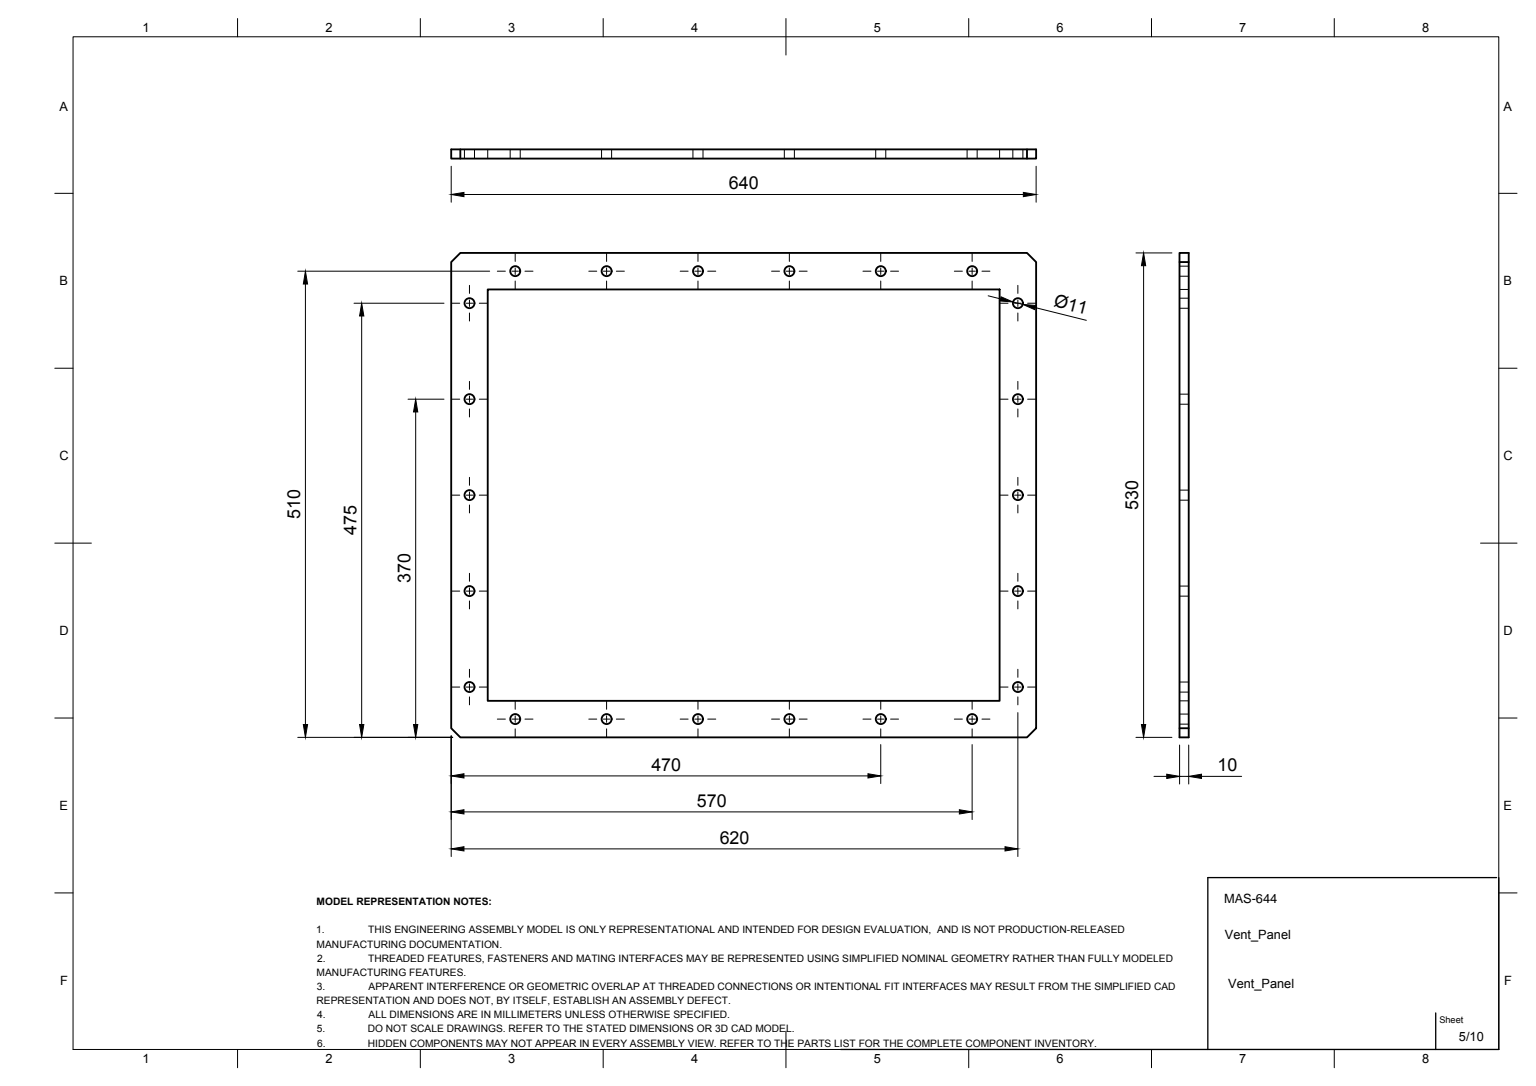
ISO-10303-21;
HEADER;
FILE_DESCRIPTION((''),'2;1');
FILE_NAME('Vent_Panel.step','2026-10-09T11:38:21-07:00',(''),(''),'','','');
FILE_SCHEMA (('AUTOMOTIVE_DESIGN { 1 0 10303 214 3 1 1 }'));
ENDSEC;
DATA;
#10=MECHANICAL_DESIGN_GEOMETRIC_PRESENTATION_REPRESENTATION('',(#61),#3619);
#45=SHAPE_REPRESENTATION_RELATIONSHIP('SRR','None',#3653,#53) ;
#53=ADVANCED_BREP_SHAPE_REPRESENTATION('',(#69),#3613) ;
#61=STYLED_ITEM('',(#3700),#69) ;
#69=MANIFOLD_SOLID_BREP('Body1',#2085) ;
#111=FACE_BOUND('',#414,.T.) ;
#112=FACE_BOUND('',#415,.T.) ;
#113=FACE_BOUND('',#416,.T.) ;
#114=FACE_BOUND('',#417,.T.) ;
#115=FACE_BOUND('',#418,.T.) ;
#116=FACE_BOUND('',#419,.T.) ;
#117=FACE_BOUND('',#420,.T.) ;
#118=FACE_BOUND('',#421,.T.) ;
#119=FACE_BOUND('',#422,.T.) ;
#120=FACE_BOUND('',#423,.T.) ;
#121=FACE_BOUND('',#424,.T.) ;
#122=FACE_BOUND('',#425,.T.) ;
#123=FACE_BOUND('',#426,.T.) ;
#124=FACE_BOUND('',#427,.T.) ;
#125=FACE_BOUND('',#428,.T.) ;
#126=FACE_BOUND('',#429,.T.) ;
#127=FACE_BOUND('',#430,.T.) ;
#128=FACE_BOUND('',#431,.T.) ;
#129=FACE_BOUND('',#432,.T.) ;
#130=FACE_BOUND('',#433,.T.) ;
#131=FACE_BOUND('',#434,.T.) ;
#132=FACE_BOUND('',#435,.T.) ;
#133=FACE_BOUND('',#436,.T.) ;
#134=FACE_BOUND('',#438,.T.) ;
#135=FACE_BOUND('',#439,.T.) ;
#136=FACE_BOUND('',#440,.T.) ;
#137=FACE_BOUND('',#441,.T.) ;
#138=FACE_BOUND('',#442,.T.) ;
#139=FACE_BOUND('',#443,.T.) ;
#140=FACE_BOUND('',#444,.T.) ;
#141=FACE_BOUND('',#445,.T.) ;
#142=FACE_BOUND('',#446,.T.) ;
#143=FACE_BOUND('',#447,.T.) ;
#144=FACE_BOUND('',#448,.T.) ;
#145=FACE_BOUND('',#449,.T.) ;
#146=FACE_BOUND('',#450,.T.) ;
#147=FACE_BOUND('',#451,.T.) ;
#148=FACE_BOUND('',#452,.T.) ;
#149=FACE_BOUND('',#453,.T.) ;
#150=FACE_BOUND('',#454,.T.) ;
#151=FACE_BOUND('',#455,.T.) ;
#152=FACE_BOUND('',#456,.T.) ;
#153=FACE_BOUND('',#457,.T.) ;
#154=FACE_BOUND('',#458,.T.) ;
#155=FACE_BOUND('',#459,.T.) ;
#156=FACE_BOUND('',#460,.T.) ;
#169=PLANE('',#2328) ;
#170=PLANE('',#2329) ;
#171=PLANE('',#2330) ;
#172=PLANE('',#2331) ;
#173=PLANE('',#2332) ;
#174=PLANE('',#2333) ;
#175=PLANE('',#2334) ;
#176=PLANE('',#2335) ;
#177=PLANE('',#2336) ;
#178=PLANE('',#2337) ;
#179=PLANE('',#2338) ;
#180=PLANE('',#2339) ;
#181=PLANE('',#2340) ;
#182=PLANE('',#2341) ;
#247=FACE_OUTER_BOUND('',#391,.T.) ;
#248=FACE_OUTER_BOUND('',#392,.T.) ;
#249=FACE_OUTER_BOUND('',#393,.T.) ;
#250=FACE_OUTER_BOUND('',#394,.T.) ;
#251=FACE_OUTER_BOUND('',#395,.T.) ;
#252=FACE_OUTER_BOUND('',#396,.T.) ;
#253=FACE_OUTER_BOUND('',#397,.T.) ;
#254=FACE_OUTER_BOUND('',#398,.T.) ;
#255=FACE_OUTER_BOUND('',#399,.T.) ;
#256=FACE_OUTER_BOUND('',#400,.T.) ;
#257=FACE_OUTER_BOUND('',#401,.T.) ;
#258=FACE_OUTER_BOUND('',#402,.T.) ;
#259=FACE_OUTER_BOUND('',#403,.T.) ;
#260=FACE_OUTER_BOUND('',#404,.T.) ;
#261=FACE_OUTER_BOUND('',#405,.T.) ;
#262=FACE_OUTER_BOUND('',#406,.T.) ;
#263=FACE_OUTER_BOUND('',#407,.T.) ;
#264=FACE_OUTER_BOUND('',#408,.T.) ;
#265=FACE_OUTER_BOUND('',#409,.T.) ;
#266=FACE_OUTER_BOUND('',#410,.T.) ;
#267=FACE_OUTER_BOUND('',#411,.T.) ;
#268=FACE_OUTER_BOUND('',#412,.T.) ;
#269=FACE_OUTER_BOUND('',#413,.T.) ;
#270=FACE_OUTER_BOUND('',#437,.T.) ;
#271=FACE_OUTER_BOUND('',#461,.T.) ;
#272=FACE_OUTER_BOUND('',#462,.T.) ;
#273=FACE_OUTER_BOUND('',#463,.T.) ;
#274=FACE_OUTER_BOUND('',#464,.T.) ;
#275=FACE_OUTER_BOUND('',#465,.T.) ;
#276=FACE_OUTER_BOUND('',#466,.T.) ;
#277=FACE_OUTER_BOUND('',#467,.T.) ;
#278=FACE_OUTER_BOUND('',#468,.T.) ;
#279=FACE_OUTER_BOUND('',#469,.T.) ;
#280=FACE_OUTER_BOUND('',#470,.T.) ;
#281=FACE_OUTER_BOUND('',#471,.T.) ;
#282=FACE_OUTER_BOUND('',#472,.T.) ;
#391=EDGE_LOOP('',(#1567,#1568,#1569,#1570)) ;
#392=EDGE_LOOP('',(#1571,#1572,#1573,#1574)) ;
#393=EDGE_LOOP('',(#1575,#1576,#1577,#1578)) ;
#394=EDGE_LOOP('',(#1579,#1580,#1581,#1582)) ;
#395=EDGE_LOOP('',(#1583,#1584,#1585,#1586)) ;
#396=EDGE_LOOP('',(#1587,#1588,#1589,#1590)) ;
#397=EDGE_LOOP('',(#1591,#1592,#1593,#1594)) ;
#398=EDGE_LOOP('',(#1595,#1596,#1597,#1598)) ;
#399=EDGE_LOOP('',(#1599,#1600,#1601,#1602)) ;
#400=EDGE_LOOP('',(#1603,#1604,#1605,#1606)) ;
#401=EDGE_LOOP('',(#1607,#1608,#1609,#1610)) ;
#402=EDGE_LOOP('',(#1611,#1612,#1613,#1614)) ;
#403=EDGE_LOOP('',(#1615,#1616,#1617,#1618)) ;
#404=EDGE_LOOP('',(#1619,#1620,#1621,#1622)) ;
#405=EDGE_LOOP('',(#1623,#1624,#1625,#1626)) ;
#406=EDGE_LOOP('',(#1627,#1628,#1629,#1630)) ;
#407=EDGE_LOOP('',(#1631,#1632,#1633,#1634)) ;
#408=EDGE_LOOP('',(#1635,#1636,#1637,#1638)) ;
#409=EDGE_LOOP('',(#1639,#1640,#1641,#1642)) ;
#410=EDGE_LOOP('',(#1643,#1644,#1645,#1646)) ;
#411=EDGE_LOOP('',(#1647,#1648,#1649,#1650)) ;
#412=EDGE_LOOP('',(#1651,#1652,#1653,#1654)) ;
#413=EDGE_LOOP('',(#1655,#1656,#1657,#1658,#1659,#1660,#1661,#1662)) ;
#414=EDGE_LOOP('',(#1663,#1664,#1665,#1666)) ;
#415=EDGE_LOOP('',(#1667)) ;
#416=EDGE_LOOP('',(#1668)) ;
#417=EDGE_LOOP('',(#1669)) ;
#418=EDGE_LOOP('',(#1670)) ;
#419=EDGE_LOOP('',(#1671)) ;
#420=EDGE_LOOP('',(#1672)) ;
#421=EDGE_LOOP('',(#1673)) ;
#422=EDGE_LOOP('',(#1674)) ;
#423=EDGE_LOOP('',(#1675)) ;
#424=EDGE_LOOP('',(#1676)) ;
#425=EDGE_LOOP('',(#1677)) ;
#426=EDGE_LOOP('',(#1678)) ;
#427=EDGE_LOOP('',(#1679)) ;
#428=EDGE_LOOP('',(#1680)) ;
#429=EDGE_LOOP('',(#1681)) ;
#430=EDGE_LOOP('',(#1682)) ;
#431=EDGE_LOOP('',(#1683)) ;
#432=EDGE_LOOP('',(#1684)) ;
#433=EDGE_LOOP('',(#1685)) ;
#434=EDGE_LOOP('',(#1686)) ;
#435=EDGE_LOOP('',(#1687)) ;
#436=EDGE_LOOP('',(#1688)) ;
#437=EDGE_LOOP('',(#1689,#1690,#1691,#1692,#1693,#1694,#1695,#1696)) ;
#438=EDGE_LOOP('',(#1697,#1698,#1699,#1700)) ;
#439=EDGE_LOOP('',(#1701)) ;
#440=EDGE_LOOP('',(#1702)) ;
#441=EDGE_LOOP('',(#1703)) ;
#442=EDGE_LOOP('',(#1704)) ;
#443=EDGE_LOOP('',(#1705)) ;
#444=EDGE_LOOP('',(#1706)) ;
#445=EDGE_LOOP('',(#1707)) ;
#446=EDGE_LOOP('',(#1708)) ;
#447=EDGE_LOOP('',(#1709)) ;
#448=EDGE_LOOP('',(#1710)) ;
#449=EDGE_LOOP('',(#1711)) ;
#450=EDGE_LOOP('',(#1712)) ;
#451=EDGE_LOOP('',(#1713)) ;
#452=EDGE_LOOP('',(#1714)) ;
#453=EDGE_LOOP('',(#1715)) ;
#454=EDGE_LOOP('',(#1716)) ;
#455=EDGE_LOOP('',(#1717)) ;
#456=EDGE_LOOP('',(#1718)) ;
#457=EDGE_LOOP('',(#1719)) ;
#458=EDGE_LOOP('',(#1720)) ;
#459=EDGE_LOOP('',(#1721)) ;
#460=EDGE_LOOP('',(#1722)) ;
#461=EDGE_LOOP('',(#1723,#1724,#1725,#1726)) ;
#462=EDGE_LOOP('',(#1727,#1728,#1729,#1730)) ;
#463=EDGE_LOOP('',(#1731,#1732,#1733,#1734)) ;
#464=EDGE_LOOP('',(#1735,#1736,#1737,#1738)) ;
#465=EDGE_LOOP('',(#1739,#1740,#1741,#1742)) ;
#466=EDGE_LOOP('',(#1743,#1744,#1745,#1746)) ;
#467=EDGE_LOOP('',(#1747,#1748,#1749,#1750)) ;
#468=EDGE_LOOP('',(#1751,#1752,#1753,#1754)) ;
#469=EDGE_LOOP('',(#1755,#1756,#1757,#1758)) ;
#470=EDGE_LOOP('',(#1759,#1760,#1761,#1762)) ;
#471=EDGE_LOOP('',(#1763,#1764,#1765,#1766)) ;
#472=EDGE_LOOP('',(#1767,#1768,#1769,#1770)) ;
#557=LINE('',#3223,#721) ;
#558=LINE('',#3229,#722) ;
#559=LINE('',#3235,#723) ;
#560=LINE('',#3241,#724) ;
#561=LINE('',#3247,#725) ;
#562=LINE('',#3253,#726) ;
#563=LINE('',#3259,#727) ;
#564=LINE('',#3265,#728) ;
#565=LINE('',#3271,#729) ;
#566=LINE('',#3277,#730) ;
#567=LINE('',#3283,#731) ;
#568=LINE('',#3289,#732) ;
#569=LINE('',#3295,#733) ;
#570=LINE('',#3301,#734) ;
#571=LINE('',#3307,#735) ;
#572=LINE('',#3313,#736) ;
#573=LINE('',#3319,#737) ;
#574=LINE('',#3325,#738) ;
#575=LINE('',#3331,#739) ;
#576=LINE('',#3337,#740) ;
#577=LINE('',#3343,#741) ;
#578=LINE('',#3349,#742) ;
#579=LINE('',#3354,#743) ;
#580=LINE('',#3356,#744) ;
#581=LINE('',#3358,#745) ;
#582=LINE('',#3360,#746) ;
#583=LINE('',#3362,#747) ;
#584=LINE('',#3364,#748) ;
#585=LINE('',#3366,#749) ;
#586=LINE('',#3367,#750) ;
#587=LINE('',#3370,#751) ;
#588=LINE('',#3372,#752) ;
#589=LINE('',#3374,#753) ;
#590=LINE('',#3375,#754) ;
#591=LINE('',#3379,#755) ;
#592=LINE('',#3381,#756) ;
#593=LINE('',#3383,#757) ;
#594=LINE('',#3385,#758) ;
#595=LINE('',#3387,#759) ;
#596=LINE('',#3389,#760) ;
#597=LINE('',#3391,#761) ;
#598=LINE('',#3392,#762) ;
#599=LINE('',#3395,#763) ;
#600=LINE('',#3397,#764) ;
#601=LINE('',#3399,#765) ;
#602=LINE('',#3400,#766) ;
#603=LINE('',#3402,#767) ;
#604=LINE('',#3403,#768) ;
#605=LINE('',#3405,#769) ;
#606=LINE('',#3407,#770) ;
#607=LINE('',#3409,#771) ;
#608=LINE('',#3411,#772) ;
#609=LINE('',#3413,#773) ;
#610=LINE('',#3415,#774) ;
#611=LINE('',#3418,#775) ;
#612=LINE('',#3419,#776) ;
#613=LINE('',#3421,#777) ;
#614=LINE('',#3423,#778) ;
#721=VECTOR('',#2623,5.50000000000002) ;
#722=VECTOR('',#2630,5.50000000000002) ;
#723=VECTOR('',#2637,5.50000000000001) ;
#724=VECTOR('',#2644,5.50000000000001) ;
#725=VECTOR('',#2651,5.50000000000001) ;
#726=VECTOR('',#2658,5.50000000000001) ;
#727=VECTOR('',#2665,5.50000000000001) ;
#728=VECTOR('',#2672,5.50000000000001) ;
#729=VECTOR('',#2679,5.50000000000002) ;
#730=VECTOR('',#2686,5.50000000000002) ;
#731=VECTOR('',#2693,5.49999999999999) ;
#732=VECTOR('',#2700,5.49999999999999) ;
#733=VECTOR('',#2707,5.49999999999999) ;
#734=VECTOR('',#2714,5.49999999999999) ;
#735=VECTOR('',#2721,5.49999999999999) ;
#736=VECTOR('',#2728,5.50000000000002) ;
#737=VECTOR('',#2735,5.50000000000001) ;
#738=VECTOR('',#2742,5.50000000000001) ;
#739=VECTOR('',#2749,5.50000000000001) ;
#740=VECTOR('',#2756,5.50000000000001) ;
#741=VECTOR('',#2763,5.50000000000001) ;
#742=VECTOR('',#2770,5.50000000000001) ;
#743=VECTOR('',#2775,1000.) ;
#744=VECTOR('',#2776,1000.) ;
#745=VECTOR('',#2777,1000.) ;
#746=VECTOR('',#2778,1000.) ;
#747=VECTOR('',#2779,1000.) ;
#748=VECTOR('',#2780,1000.) ;
#749=VECTOR('',#2781,1000.) ;
#750=VECTOR('',#2782,1000.) ;
#751=VECTOR('',#2783,1000.) ;
#752=VECTOR('',#2784,1000.) ;
#753=VECTOR('',#2785,1000.) ;
#754=VECTOR('',#2786,1000.) ;
#755=VECTOR('',#2789,1000.) ;
#756=VECTOR('',#2790,1000.) ;
#757=VECTOR('',#2791,1000.) ;
#758=VECTOR('',#2792,1000.) ;
#759=VECTOR('',#2793,1000.) ;
#760=VECTOR('',#2794,1000.) ;
#761=VECTOR('',#2795,1000.) ;
#762=VECTOR('',#2796,1000.) ;
#763=VECTOR('',#2797,1000.) ;
#764=VECTOR('',#2798,1000.) ;
#765=VECTOR('',#2799,1000.) ;
#766=VECTOR('',#2800,1000.) ;
#767=VECTOR('',#2803,1000.) ;
#768=VECTOR('',#2804,1000.) ;
#769=VECTOR('',#2807,1000.) ;
#770=VECTOR('',#2810,1000.) ;
#771=VECTOR('',#2813,1000.) ;
#772=VECTOR('',#2816,1000.) ;
#773=VECTOR('',#2819,1000.) ;
#774=VECTOR('',#2822,1000.) ;
#775=VECTOR('',#2827,1000.) ;
#776=VECTOR('',#2828,1000.) ;
#777=VECTOR('',#2831,1000.) ;
#778=VECTOR('',#2834,1000.) ;
#883=CIRCLE('',#2263,5.50000000000002) ;
#884=CIRCLE('',#2264,5.50000000000002) ;
#885=CIRCLE('',#2266,5.50000000000002) ;
#886=CIRCLE('',#2267,5.50000000000002) ;
#887=CIRCLE('',#2269,5.50000000000001) ;
#888=CIRCLE('',#2270,5.50000000000001) ;
#889=CIRCLE('',#2272,5.50000000000001) ;
#890=CIRCLE('',#2273,5.50000000000001) ;
#891=CIRCLE('',#2275,5.50000000000001) ;
#892=CIRCLE('',#2276,5.50000000000001) ;
#893=CIRCLE('',#2278,5.50000000000001) ;
#894=CIRCLE('',#2279,5.50000000000001) ;
#895=CIRCLE('',#2281,5.50000000000001) ;
#896=CIRCLE('',#2282,5.50000000000001) ;
#897=CIRCLE('',#2284,5.50000000000001) ;
#898=CIRCLE('',#2285,5.50000000000001) ;
#899=CIRCLE('',#2287,5.50000000000002) ;
#900=CIRCLE('',#2288,5.50000000000002) ;
#901=CIRCLE('',#2290,5.50000000000002) ;
#902=CIRCLE('',#2291,5.50000000000002) ;
#903=CIRCLE('',#2293,5.49999999999999) ;
#904=CIRCLE('',#2294,5.49999999999999) ;
#905=CIRCLE('',#2296,5.49999999999999) ;
#906=CIRCLE('',#2297,5.49999999999999) ;
#907=CIRCLE('',#2299,5.49999999999999) ;
#908=CIRCLE('',#2300,5.49999999999999) ;
#909=CIRCLE('',#2302,5.49999999999999) ;
#910=CIRCLE('',#2303,5.49999999999999) ;
#911=CIRCLE('',#2305,5.49999999999999) ;
#912=CIRCLE('',#2306,5.49999999999999) ;
#913=CIRCLE('',#2308,5.50000000000002) ;
#914=CIRCLE('',#2309,5.50000000000002) ;
#915=CIRCLE('',#2311,5.50000000000001) ;
#916=CIRCLE('',#2312,5.50000000000001) ;
#917=CIRCLE('',#2314,5.50000000000001) ;
#918=CIRCLE('',#2315,5.50000000000001) ;
#919=CIRCLE('',#2317,5.50000000000001) ;
#920=CIRCLE('',#2318,5.50000000000001) ;
#921=CIRCLE('',#2320,5.50000000000001) ;
#922=CIRCLE('',#2321,5.50000000000001) ;
#923=CIRCLE('',#2323,5.50000000000001) ;
#924=CIRCLE('',#2324,5.50000000000001) ;
#925=CIRCLE('',#2326,5.50000000000001) ;
#926=CIRCLE('',#2327,5.50000000000001) ;
#1003=VERTEX_POINT('',#3220) ;
#1004=VERTEX_POINT('',#3222) ;
#1005=VERTEX_POINT('',#3226) ;
#1006=VERTEX_POINT('',#3228) ;
#1007=VERTEX_POINT('',#3232) ;
#1008=VERTEX_POINT('',#3234) ;
#1009=VERTEX_POINT('',#3238) ;
#1010=VERTEX_POINT('',#3240) ;
#1011=VERTEX_POINT('',#3244) ;
#1012=VERTEX_POINT('',#3246) ;
#1013=VERTEX_POINT('',#3250) ;
#1014=VERTEX_POINT('',#3252) ;
#1015=VERTEX_POINT('',#3256) ;
#1016=VERTEX_POINT('',#3258) ;
#1017=VERTEX_POINT('',#3262) ;
#1018=VERTEX_POINT('',#3264) ;
#1019=VERTEX_POINT('',#3268) ;
#1020=VERTEX_POINT('',#3270) ;
#1021=VERTEX_POINT('',#3274) ;
#1022=VERTEX_POINT('',#3276) ;
#1023=VERTEX_POINT('',#3280) ;
#1024=VERTEX_POINT('',#3282) ;
#1025=VERTEX_POINT('',#3286) ;
#1026=VERTEX_POINT('',#3288) ;
#1027=VERTEX_POINT('',#3292) ;
#1028=VERTEX_POINT('',#3294) ;
#1029=VERTEX_POINT('',#3298) ;
#1030=VERTEX_POINT('',#3300) ;
#1031=VERTEX_POINT('',#3304) ;
#1032=VERTEX_POINT('',#3306) ;
#1033=VERTEX_POINT('',#3310) ;
#1034=VERTEX_POINT('',#3312) ;
#1035=VERTEX_POINT('',#3316) ;
#1036=VERTEX_POINT('',#3318) ;
#1037=VERTEX_POINT('',#3322) ;
#1038=VERTEX_POINT('',#3324) ;
#1039=VERTEX_POINT('',#3328) ;
#1040=VERTEX_POINT('',#3330) ;
#1041=VERTEX_POINT('',#3334) ;
#1042=VERTEX_POINT('',#3336) ;
#1043=VERTEX_POINT('',#3340) ;
#1044=VERTEX_POINT('',#3342) ;
#1045=VERTEX_POINT('',#3346) ;
#1046=VERTEX_POINT('',#3348) ;
#1047=VERTEX_POINT('',#3352) ;
#1048=VERTEX_POINT('',#3353) ;
#1049=VERTEX_POINT('',#3355) ;
#1050=VERTEX_POINT('',#3357) ;
#1051=VERTEX_POINT('',#3359) ;
#1052=VERTEX_POINT('',#3361) ;
#1053=VERTEX_POINT('',#3363) ;
#1054=VERTEX_POINT('',#3365) ;
#1055=VERTEX_POINT('',#3368) ;
#1056=VERTEX_POINT('',#3369) ;
#1057=VERTEX_POINT('',#3371) ;
#1058=VERTEX_POINT('',#3373) ;
#1059=VERTEX_POINT('',#3377) ;
#1060=VERTEX_POINT('',#3378) ;
#1061=VERTEX_POINT('',#3380) ;
#1062=VERTEX_POINT('',#3382) ;
#1063=VERTEX_POINT('',#3384) ;
#1064=VERTEX_POINT('',#3386) ;
#1065=VERTEX_POINT('',#3388) ;
#1066=VERTEX_POINT('',#3390) ;
#1067=VERTEX_POINT('',#3393) ;
#1068=VERTEX_POINT('',#3394) ;
#1069=VERTEX_POINT('',#3396) ;
#1070=VERTEX_POINT('',#3398) ;
#1209=EDGE_CURVE('',#1003,#1003,#883,.T.) ;
#1210=EDGE_CURVE('',#1003,#1004,#557,.T.) ;
#1211=EDGE_CURVE('',#1004,#1004,#884,.T.) ;
#1212=EDGE_CURVE('',#1005,#1005,#885,.T.) ;
#1213=EDGE_CURVE('',#1005,#1006,#558,.T.) ;
#1214=EDGE_CURVE('',#1006,#1006,#886,.T.) ;
#1215=EDGE_CURVE('',#1007,#1007,#887,.T.) ;
#1216=EDGE_CURVE('',#1007,#1008,#559,.T.) ;
#1217=EDGE_CURVE('',#1008,#1008,#888,.T.) ;
#1218=EDGE_CURVE('',#1009,#1009,#889,.T.) ;
#1219=EDGE_CURVE('',#1009,#1010,#560,.T.) ;
#1220=EDGE_CURVE('',#1010,#1010,#890,.T.) ;
#1221=EDGE_CURVE('',#1011,#1011,#891,.T.) ;
#1222=EDGE_CURVE('',#1011,#1012,#561,.T.) ;
#1223=EDGE_CURVE('',#1012,#1012,#892,.T.) ;
#1224=EDGE_CURVE('',#1013,#1013,#893,.T.) ;
#1225=EDGE_CURVE('',#1013,#1014,#562,.T.) ;
#1226=EDGE_CURVE('',#1014,#1014,#894,.T.) ;
#1227=EDGE_CURVE('',#1015,#1015,#895,.T.) ;
#1228=EDGE_CURVE('',#1015,#1016,#563,.T.) ;
#1229=EDGE_CURVE('',#1016,#1016,#896,.T.) ;
#1230=EDGE_CURVE('',#1017,#1017,#897,.T.) ;
#1231=EDGE_CURVE('',#1017,#1018,#564,.T.) ;
#1232=EDGE_CURVE('',#1018,#1018,#898,.T.) ;
#1233=EDGE_CURVE('',#1019,#1019,#899,.T.) ;
#1234=EDGE_CURVE('',#1019,#1020,#565,.T.) ;
#1235=EDGE_CURVE('',#1020,#1020,#900,.T.) ;
#1236=EDGE_CURVE('',#1021,#1021,#901,.T.) ;
#1237=EDGE_CURVE('',#1021,#1022,#566,.T.) ;
#1238=EDGE_CURVE('',#1022,#1022,#902,.T.) ;
#1239=EDGE_CURVE('',#1023,#1023,#903,.T.) ;
#1240=EDGE_CURVE('',#1023,#1024,#567,.T.) ;
#1241=EDGE_CURVE('',#1024,#1024,#904,.T.) ;
#1242=EDGE_CURVE('',#1025,#1025,#905,.T.) ;
#1243=EDGE_CURVE('',#1025,#1026,#568,.T.) ;
#1244=EDGE_CURVE('',#1026,#1026,#906,.T.) ;
#1245=EDGE_CURVE('',#1027,#1027,#907,.T.) ;
#1246=EDGE_CURVE('',#1027,#1028,#569,.T.) ;
#1247=EDGE_CURVE('',#1028,#1028,#908,.T.) ;
#1248=EDGE_CURVE('',#1029,#1029,#909,.T.) ;
#1249=EDGE_CURVE('',#1029,#1030,#570,.T.) ;
#1250=EDGE_CURVE('',#1030,#1030,#910,.T.) ;
#1251=EDGE_CURVE('',#1031,#1031,#911,.T.) ;
#1252=EDGE_CURVE('',#1031,#1032,#571,.T.) ;
#1253=EDGE_CURVE('',#1032,#1032,#912,.T.) ;
#1254=EDGE_CURVE('',#1033,#1033,#913,.T.) ;
#1255=EDGE_CURVE('',#1033,#1034,#572,.T.) ;
#1256=EDGE_CURVE('',#1034,#1034,#914,.T.) ;
#1257=EDGE_CURVE('',#1035,#1035,#915,.T.) ;
#1258=EDGE_CURVE('',#1035,#1036,#573,.T.) ;
#1259=EDGE_CURVE('',#1036,#1036,#916,.T.) ;
#1260=EDGE_CURVE('',#1037,#1037,#917,.T.) ;
#1261=EDGE_CURVE('',#1037,#1038,#574,.T.) ;
#1262=EDGE_CURVE('',#1038,#1038,#918,.T.) ;
#1263=EDGE_CURVE('',#1039,#1039,#919,.T.) ;
#1264=EDGE_CURVE('',#1039,#1040,#575,.T.) ;
#1265=EDGE_CURVE('',#1040,#1040,#920,.T.) ;
#1266=EDGE_CURVE('',#1041,#1041,#921,.T.) ;
#1267=EDGE_CURVE('',#1041,#1042,#576,.T.) ;
#1268=EDGE_CURVE('',#1042,#1042,#922,.T.) ;
#1269=EDGE_CURVE('',#1043,#1043,#923,.T.) ;
#1270=EDGE_CURVE('',#1043,#1044,#577,.T.) ;
#1271=EDGE_CURVE('',#1044,#1044,#924,.T.) ;
#1272=EDGE_CURVE('',#1045,#1045,#925,.T.) ;
#1273=EDGE_CURVE('',#1045,#1046,#578,.T.) ;
#1274=EDGE_CURVE('',#1046,#1046,#926,.T.) ;
#1275=EDGE_CURVE('',#1047,#1048,#579,.T.) ;
#1276=EDGE_CURVE('',#1048,#1049,#580,.T.) ;
#1277=EDGE_CURVE('',#1049,#1050,#581,.T.) ;
#1278=EDGE_CURVE('',#1050,#1051,#582,.T.) ;
#1279=EDGE_CURVE('',#1051,#1052,#583,.T.) ;
#1280=EDGE_CURVE('',#1052,#1053,#584,.T.) ;
#1281=EDGE_CURVE('',#1053,#1054,#585,.T.) ;
#1282=EDGE_CURVE('',#1054,#1047,#586,.T.) ;
#1283=EDGE_CURVE('',#1055,#1056,#587,.T.) ;
#1284=EDGE_CURVE('',#1057,#1055,#588,.T.) ;
#1285=EDGE_CURVE('',#1058,#1057,#589,.T.) ;
#1286=EDGE_CURVE('',#1056,#1058,#590,.T.) ;
#1287=EDGE_CURVE('',#1059,#1060,#591,.T.) ;
#1288=EDGE_CURVE('',#1061,#1059,#592,.T.) ;
#1289=EDGE_CURVE('',#1062,#1061,#593,.T.) ;
#1290=EDGE_CURVE('',#1063,#1062,#594,.T.) ;
#1291=EDGE_CURVE('',#1064,#1063,#595,.T.) ;
#1292=EDGE_CURVE('',#1065,#1064,#596,.T.) ;
#1293=EDGE_CURVE('',#1066,#1065,#597,.T.) ;
#1294=EDGE_CURVE('',#1060,#1066,#598,.T.) ;
#1295=EDGE_CURVE('',#1067,#1068,#599,.T.) ;
#1296=EDGE_CURVE('',#1068,#1069,#600,.T.) ;
#1297=EDGE_CURVE('',#1069,#1070,#601,.T.) ;
#1298=EDGE_CURVE('',#1070,#1067,#602,.T.) ;
#1299=EDGE_CURVE('',#1048,#1060,#603,.T.) ;
#1300=EDGE_CURVE('',#1047,#1059,#604,.T.) ;
#1301=EDGE_CURVE('',#1049,#1066,#605,.T.) ;
#1302=EDGE_CURVE('',#1050,#1065,#606,.T.) ;
#1303=EDGE_CURVE('',#1051,#1064,#607,.T.) ;
#1304=EDGE_CURVE('',#1052,#1063,#608,.T.) ;
#1305=EDGE_CURVE('',#1053,#1062,#609,.T.) ;
#1306=EDGE_CURVE('',#1054,#1061,#610,.T.) ;
#1307=EDGE_CURVE('',#1057,#1067,#611,.T.) ;
#1308=EDGE_CURVE('',#1055,#1068,#612,.T.) ;
#1309=EDGE_CURVE('',#1056,#1069,#613,.T.) ;
#1310=EDGE_CURVE('',#1058,#1070,#614,.T.) ;
#1567=ORIENTED_EDGE('',*,*,#1209,.T.) ;
#1568=ORIENTED_EDGE('',*,*,#1210,.T.) ;
#1569=ORIENTED_EDGE('',*,*,#1211,.F.) ;
#1570=ORIENTED_EDGE('',*,*,#1210,.F.) ;
#1571=ORIENTED_EDGE('',*,*,#1212,.T.) ;
#1572=ORIENTED_EDGE('',*,*,#1213,.T.) ;
#1573=ORIENTED_EDGE('',*,*,#1214,.F.) ;
#1574=ORIENTED_EDGE('',*,*,#1213,.F.) ;
#1575=ORIENTED_EDGE('',*,*,#1215,.T.) ;
#1576=ORIENTED_EDGE('',*,*,#1216,.T.) ;
#1577=ORIENTED_EDGE('',*,*,#1217,.F.) ;
#1578=ORIENTED_EDGE('',*,*,#1216,.F.) ;
#1579=ORIENTED_EDGE('',*,*,#1218,.T.) ;
#1580=ORIENTED_EDGE('',*,*,#1219,.T.) ;
#1581=ORIENTED_EDGE('',*,*,#1220,.F.) ;
#1582=ORIENTED_EDGE('',*,*,#1219,.F.) ;
#1583=ORIENTED_EDGE('',*,*,#1221,.T.) ;
#1584=ORIENTED_EDGE('',*,*,#1222,.T.) ;
#1585=ORIENTED_EDGE('',*,*,#1223,.F.) ;
#1586=ORIENTED_EDGE('',*,*,#1222,.F.) ;
#1587=ORIENTED_EDGE('',*,*,#1224,.T.) ;
#1588=ORIENTED_EDGE('',*,*,#1225,.T.) ;
#1589=ORIENTED_EDGE('',*,*,#1226,.F.) ;
#1590=ORIENTED_EDGE('',*,*,#1225,.F.) ;
#1591=ORIENTED_EDGE('',*,*,#1227,.T.) ;
#1592=ORIENTED_EDGE('',*,*,#1228,.T.) ;
#1593=ORIENTED_EDGE('',*,*,#1229,.F.) ;
#1594=ORIENTED_EDGE('',*,*,#1228,.F.) ;
#1595=ORIENTED_EDGE('',*,*,#1230,.T.) ;
#1596=ORIENTED_EDGE('',*,*,#1231,.T.) ;
#1597=ORIENTED_EDGE('',*,*,#1232,.F.) ;
#1598=ORIENTED_EDGE('',*,*,#1231,.F.) ;
#1599=ORIENTED_EDGE('',*,*,#1233,.T.) ;
#1600=ORIENTED_EDGE('',*,*,#1234,.T.) ;
#1601=ORIENTED_EDGE('',*,*,#1235,.F.) ;
#1602=ORIENTED_EDGE('',*,*,#1234,.F.) ;
#1603=ORIENTED_EDGE('',*,*,#1236,.T.) ;
#1604=ORIENTED_EDGE('',*,*,#1237,.T.) ;
#1605=ORIENTED_EDGE('',*,*,#1238,.F.) ;
#1606=ORIENTED_EDGE('',*,*,#1237,.F.) ;
#1607=ORIENTED_EDGE('',*,*,#1239,.T.) ;
#1608=ORIENTED_EDGE('',*,*,#1240,.T.) ;
#1609=ORIENTED_EDGE('',*,*,#1241,.F.) ;
#1610=ORIENTED_EDGE('',*,*,#1240,.F.) ;
#1611=ORIENTED_EDGE('',*,*,#1242,.T.) ;
#1612=ORIENTED_EDGE('',*,*,#1243,.T.) ;
#1613=ORIENTED_EDGE('',*,*,#1244,.F.) ;
#1614=ORIENTED_EDGE('',*,*,#1243,.F.) ;
#1615=ORIENTED_EDGE('',*,*,#1245,.T.) ;
#1616=ORIENTED_EDGE('',*,*,#1246,.T.) ;
#1617=ORIENTED_EDGE('',*,*,#1247,.F.) ;
#1618=ORIENTED_EDGE('',*,*,#1246,.F.) ;
#1619=ORIENTED_EDGE('',*,*,#1248,.T.) ;
#1620=ORIENTED_EDGE('',*,*,#1249,.T.) ;
#1621=ORIENTED_EDGE('',*,*,#1250,.F.) ;
#1622=ORIENTED_EDGE('',*,*,#1249,.F.) ;
#1623=ORIENTED_EDGE('',*,*,#1251,.T.) ;
#1624=ORIENTED_EDGE('',*,*,#1252,.T.) ;
#1625=ORIENTED_EDGE('',*,*,#1253,.F.) ;
#1626=ORIENTED_EDGE('',*,*,#1252,.F.) ;
#1627=ORIENTED_EDGE('',*,*,#1254,.T.) ;
#1628=ORIENTED_EDGE('',*,*,#1255,.T.) ;
#1629=ORIENTED_EDGE('',*,*,#1256,.F.) ;
#1630=ORIENTED_EDGE('',*,*,#1255,.F.) ;
#1631=ORIENTED_EDGE('',*,*,#1257,.T.) ;
#1632=ORIENTED_EDGE('',*,*,#1258,.T.) ;
#1633=ORIENTED_EDGE('',*,*,#1259,.F.) ;
#1634=ORIENTED_EDGE('',*,*,#1258,.F.) ;
#1635=ORIENTED_EDGE('',*,*,#1260,.T.) ;
#1636=ORIENTED_EDGE('',*,*,#1261,.T.) ;
#1637=ORIENTED_EDGE('',*,*,#1262,.F.) ;
#1638=ORIENTED_EDGE('',*,*,#1261,.F.) ;
#1639=ORIENTED_EDGE('',*,*,#1263,.T.) ;
#1640=ORIENTED_EDGE('',*,*,#1264,.T.) ;
#1641=ORIENTED_EDGE('',*,*,#1265,.F.) ;
#1642=ORIENTED_EDGE('',*,*,#1264,.F.) ;
#1643=ORIENTED_EDGE('',*,*,#1266,.T.) ;
#1644=ORIENTED_EDGE('',*,*,#1267,.T.) ;
#1645=ORIENTED_EDGE('',*,*,#1268,.F.) ;
#1646=ORIENTED_EDGE('',*,*,#1267,.F.) ;
#1647=ORIENTED_EDGE('',*,*,#1269,.T.) ;
#1648=ORIENTED_EDGE('',*,*,#1270,.T.) ;
#1649=ORIENTED_EDGE('',*,*,#1271,.F.) ;
#1650=ORIENTED_EDGE('',*,*,#1270,.F.) ;
#1651=ORIENTED_EDGE('',*,*,#1272,.T.) ;
#1652=ORIENTED_EDGE('',*,*,#1273,.T.) ;
#1653=ORIENTED_EDGE('',*,*,#1274,.F.) ;
#1654=ORIENTED_EDGE('',*,*,#1273,.F.) ;
#1655=ORIENTED_EDGE('',*,*,#1275,.T.) ;
#1656=ORIENTED_EDGE('',*,*,#1276,.T.) ;
#1657=ORIENTED_EDGE('',*,*,#1277,.T.) ;
#1658=ORIENTED_EDGE('',*,*,#1278,.T.) ;
#1659=ORIENTED_EDGE('',*,*,#1279,.T.) ;
#1660=ORIENTED_EDGE('',*,*,#1280,.T.) ;
#1661=ORIENTED_EDGE('',*,*,#1281,.T.) ;
#1662=ORIENTED_EDGE('',*,*,#1282,.T.) ;
#1663=ORIENTED_EDGE('',*,*,#1283,.F.) ;
#1664=ORIENTED_EDGE('',*,*,#1284,.F.) ;
#1665=ORIENTED_EDGE('',*,*,#1285,.F.) ;
#1666=ORIENTED_EDGE('',*,*,#1286,.F.) ;
#1667=ORIENTED_EDGE('',*,*,#1269,.F.) ;
#1668=ORIENTED_EDGE('',*,*,#1263,.F.) ;
#1669=ORIENTED_EDGE('',*,*,#1257,.F.) ;
#1670=ORIENTED_EDGE('',*,*,#1251,.F.) ;
#1671=ORIENTED_EDGE('',*,*,#1245,.F.) ;
#1672=ORIENTED_EDGE('',*,*,#1239,.F.) ;
#1673=ORIENTED_EDGE('',*,*,#1233,.F.) ;
#1674=ORIENTED_EDGE('',*,*,#1227,.F.) ;
#1675=ORIENTED_EDGE('',*,*,#1221,.F.) ;
#1676=ORIENTED_EDGE('',*,*,#1215,.F.) ;
#1677=ORIENTED_EDGE('',*,*,#1209,.F.) ;
#1678=ORIENTED_EDGE('',*,*,#1212,.F.) ;
#1679=ORIENTED_EDGE('',*,*,#1218,.F.) ;
#1680=ORIENTED_EDGE('',*,*,#1224,.F.) ;
#1681=ORIENTED_EDGE('',*,*,#1230,.F.) ;
#1682=ORIENTED_EDGE('',*,*,#1236,.F.) ;
#1683=ORIENTED_EDGE('',*,*,#1242,.F.) ;
#1684=ORIENTED_EDGE('',*,*,#1248,.F.) ;
#1685=ORIENTED_EDGE('',*,*,#1254,.F.) ;
#1686=ORIENTED_EDGE('',*,*,#1260,.F.) ;
#1687=ORIENTED_EDGE('',*,*,#1266,.F.) ;
#1688=ORIENTED_EDGE('',*,*,#1272,.F.) ;
#1689=ORIENTED_EDGE('',*,*,#1287,.F.) ;
#1690=ORIENTED_EDGE('',*,*,#1288,.F.) ;
#1691=ORIENTED_EDGE('',*,*,#1289,.F.) ;
#1692=ORIENTED_EDGE('',*,*,#1290,.F.) ;
#1693=ORIENTED_EDGE('',*,*,#1291,.F.) ;
#1694=ORIENTED_EDGE('',*,*,#1292,.F.) ;
#1695=ORIENTED_EDGE('',*,*,#1293,.F.) ;
#1696=ORIENTED_EDGE('',*,*,#1294,.F.) ;
#1697=ORIENTED_EDGE('',*,*,#1295,.T.) ;
#1698=ORIENTED_EDGE('',*,*,#1296,.T.) ;
#1699=ORIENTED_EDGE('',*,*,#1297,.T.) ;
#1700=ORIENTED_EDGE('',*,*,#1298,.T.) ;
#1701=ORIENTED_EDGE('',*,*,#1274,.T.) ;
#1702=ORIENTED_EDGE('',*,*,#1271,.T.) ;
#1703=ORIENTED_EDGE('',*,*,#1268,.T.) ;
#1704=ORIENTED_EDGE('',*,*,#1265,.T.) ;
#1705=ORIENTED_EDGE('',*,*,#1262,.T.) ;
#1706=ORIENTED_EDGE('',*,*,#1259,.T.) ;
#1707=ORIENTED_EDGE('',*,*,#1256,.T.) ;
#1708=ORIENTED_EDGE('',*,*,#1253,.T.) ;
#1709=ORIENTED_EDGE('',*,*,#1250,.T.) ;
#1710=ORIENTED_EDGE('',*,*,#1247,.T.) ;
#1711=ORIENTED_EDGE('',*,*,#1244,.T.) ;
#1712=ORIENTED_EDGE('',*,*,#1241,.T.) ;
#1713=ORIENTED_EDGE('',*,*,#1238,.T.) ;
#1714=ORIENTED_EDGE('',*,*,#1235,.T.) ;
#1715=ORIENTED_EDGE('',*,*,#1232,.T.) ;
#1716=ORIENTED_EDGE('',*,*,#1229,.T.) ;
#1717=ORIENTED_EDGE('',*,*,#1226,.T.) ;
#1718=ORIENTED_EDGE('',*,*,#1223,.T.) ;
#1719=ORIENTED_EDGE('',*,*,#1220,.T.) ;
#1720=ORIENTED_EDGE('',*,*,#1217,.T.) ;
#1721=ORIENTED_EDGE('',*,*,#1214,.T.) ;
#1722=ORIENTED_EDGE('',*,*,#1211,.T.) ;
#1723=ORIENTED_EDGE('',*,*,#1287,.T.) ;
#1724=ORIENTED_EDGE('',*,*,#1299,.F.) ;
#1725=ORIENTED_EDGE('',*,*,#1275,.F.) ;
#1726=ORIENTED_EDGE('',*,*,#1300,.T.) ;
#1727=ORIENTED_EDGE('',*,*,#1294,.T.) ;
#1728=ORIENTED_EDGE('',*,*,#1301,.F.) ;
#1729=ORIENTED_EDGE('',*,*,#1276,.F.) ;
#1730=ORIENTED_EDGE('',*,*,#1299,.T.) ;
#1731=ORIENTED_EDGE('',*,*,#1293,.T.) ;
#1732=ORIENTED_EDGE('',*,*,#1302,.F.) ;
#1733=ORIENTED_EDGE('',*,*,#1277,.F.) ;
#1734=ORIENTED_EDGE('',*,*,#1301,.T.) ;
#1735=ORIENTED_EDGE('',*,*,#1292,.T.) ;
#1736=ORIENTED_EDGE('',*,*,#1303,.F.) ;
#1737=ORIENTED_EDGE('',*,*,#1278,.F.) ;
#1738=ORIENTED_EDGE('',*,*,#1302,.T.) ;
#1739=ORIENTED_EDGE('',*,*,#1291,.T.) ;
#1740=ORIENTED_EDGE('',*,*,#1304,.F.) ;
#1741=ORIENTED_EDGE('',*,*,#1279,.F.) ;
#1742=ORIENTED_EDGE('',*,*,#1303,.T.) ;
#1743=ORIENTED_EDGE('',*,*,#1290,.T.) ;
#1744=ORIENTED_EDGE('',*,*,#1305,.F.) ;
#1745=ORIENTED_EDGE('',*,*,#1280,.F.) ;
#1746=ORIENTED_EDGE('',*,*,#1304,.T.) ;
#1747=ORIENTED_EDGE('',*,*,#1289,.T.) ;
#1748=ORIENTED_EDGE('',*,*,#1306,.F.) ;
#1749=ORIENTED_EDGE('',*,*,#1281,.F.) ;
#1750=ORIENTED_EDGE('',*,*,#1305,.T.) ;
#1751=ORIENTED_EDGE('',*,*,#1288,.T.) ;
#1752=ORIENTED_EDGE('',*,*,#1300,.F.) ;
#1753=ORIENTED_EDGE('',*,*,#1282,.F.) ;
#1754=ORIENTED_EDGE('',*,*,#1306,.T.) ;
#1755=ORIENTED_EDGE('',*,*,#1295,.F.) ;
#1756=ORIENTED_EDGE('',*,*,#1307,.F.) ;
#1757=ORIENTED_EDGE('',*,*,#1284,.T.) ;
#1758=ORIENTED_EDGE('',*,*,#1308,.T.) ;
#1759=ORIENTED_EDGE('',*,*,#1296,.F.) ;
#1760=ORIENTED_EDGE('',*,*,#1308,.F.) ;
#1761=ORIENTED_EDGE('',*,*,#1283,.T.) ;
#1762=ORIENTED_EDGE('',*,*,#1309,.T.) ;
#1763=ORIENTED_EDGE('',*,*,#1297,.F.) ;
#1764=ORIENTED_EDGE('',*,*,#1309,.F.) ;
#1765=ORIENTED_EDGE('',*,*,#1286,.T.) ;
#1766=ORIENTED_EDGE('',*,*,#1310,.T.) ;
#1767=ORIENTED_EDGE('',*,*,#1298,.F.) ;
#1768=ORIENTED_EDGE('',*,*,#1310,.F.) ;
#1769=ORIENTED_EDGE('',*,*,#1285,.T.) ;
#1770=ORIENTED_EDGE('',*,*,#1307,.T.) ;
#1945=CYLINDRICAL_SURFACE('',#2262,5.50000000000002) ;
#1946=CYLINDRICAL_SURFACE('',#2265,5.50000000000002) ;
#1947=CYLINDRICAL_SURFACE('',#2268,5.50000000000001) ;
#1948=CYLINDRICAL_SURFACE('',#2271,5.50000000000001) ;
#1949=CYLINDRICAL_SURFACE('',#2274,5.50000000000001) ;
#1950=CYLINDRICAL_SURFACE('',#2277,5.50000000000001) ;
#1951=CYLINDRICAL_SURFACE('',#2280,5.50000000000001) ;
#1952=CYLINDRICAL_SURFACE('',#2283,5.50000000000001) ;
#1953=CYLINDRICAL_SURFACE('',#2286,5.50000000000002) ;
#1954=CYLINDRICAL_SURFACE('',#2289,5.50000000000002) ;
#1955=CYLINDRICAL_SURFACE('',#2292,5.49999999999999) ;
#1956=CYLINDRICAL_SURFACE('',#2295,5.49999999999999) ;
#1957=CYLINDRICAL_SURFACE('',#2298,5.49999999999999) ;
#1958=CYLINDRICAL_SURFACE('',#2301,5.49999999999999) ;
#1959=CYLINDRICAL_SURFACE('',#2304,5.49999999999999) ;
#1960=CYLINDRICAL_SURFACE('',#2307,5.50000000000002) ;
#1961=CYLINDRICAL_SURFACE('',#2310,5.50000000000001) ;
#1962=CYLINDRICAL_SURFACE('',#2313,5.50000000000001) ;
#1963=CYLINDRICAL_SURFACE('',#2316,5.50000000000001) ;
#1964=CYLINDRICAL_SURFACE('',#2319,5.50000000000001) ;
#1965=CYLINDRICAL_SURFACE('',#2322,5.50000000000001) ;
#1966=CYLINDRICAL_SURFACE('',#2325,5.50000000000001) ;
#2009=ADVANCED_FACE('',(#247),#1945,.F.) ;
#2010=ADVANCED_FACE('',(#248),#1946,.F.) ;
#2011=ADVANCED_FACE('',(#249),#1947,.F.) ;
#2012=ADVANCED_FACE('',(#250),#1948,.F.) ;
#2013=ADVANCED_FACE('',(#251),#1949,.F.) ;
#2014=ADVANCED_FACE('',(#252),#1950,.F.) ;
#2015=ADVANCED_FACE('',(#253),#1951,.F.) ;
#2016=ADVANCED_FACE('',(#254),#1952,.F.) ;
#2017=ADVANCED_FACE('',(#255),#1953,.F.) ;
#2018=ADVANCED_FACE('',(#256),#1954,.F.) ;
#2019=ADVANCED_FACE('',(#257),#1955,.F.) ;
#2020=ADVANCED_FACE('',(#258),#1956,.F.) ;
#2021=ADVANCED_FACE('',(#259),#1957,.F.) ;
#2022=ADVANCED_FACE('',(#260),#1958,.F.) ;
#2023=ADVANCED_FACE('',(#261),#1959,.F.) ;
#2024=ADVANCED_FACE('',(#262),#1960,.F.) ;
#2025=ADVANCED_FACE('',(#263),#1961,.F.) ;
#2026=ADVANCED_FACE('',(#264),#1962,.F.) ;
#2027=ADVANCED_FACE('',(#265),#1963,.F.) ;
#2028=ADVANCED_FACE('',(#266),#1964,.F.) ;
#2029=ADVANCED_FACE('',(#267),#1965,.F.) ;
#2030=ADVANCED_FACE('',(#268),#1966,.F.) ;
#2031=ADVANCED_FACE('',(#269,#111,#112,#113,#114,#115,#116,#117,#118,#119,
#120,#121,#122,#123,#124,#125,#126,#127,#128,#129,#130,#131,#132,#133),
#169,.T.) ;
#2032=ADVANCED_FACE('',(#270,#134,#135,#136,#137,#138,#139,#140,#141,#142,
#143,#144,#145,#146,#147,#148,#149,#150,#151,#152,#153,#154,#155,#156),
#170,.F.) ;
#2033=ADVANCED_FACE('',(#271),#171,.F.) ;
#2034=ADVANCED_FACE('',(#272),#172,.F.) ;
#2035=ADVANCED_FACE('',(#273),#173,.F.) ;
#2036=ADVANCED_FACE('',(#274),#174,.F.) ;
#2037=ADVANCED_FACE('',(#275),#175,.F.) ;
#2038=ADVANCED_FACE('',(#276),#176,.F.) ;
#2039=ADVANCED_FACE('',(#277),#177,.F.) ;
#2040=ADVANCED_FACE('',(#278),#178,.F.) ;
#2041=ADVANCED_FACE('',(#279),#179,.T.) ;
#2042=ADVANCED_FACE('',(#280),#180,.T.) ;
#2043=ADVANCED_FACE('',(#281),#181,.T.) ;
#2044=ADVANCED_FACE('',(#282),#182,.T.) ;
#2085=CLOSED_SHELL('',(#2009,#2010,#2011,#2012,#2013,#2014,#2015,#2016,
#2017,#2018,#2019,#2020,#2021,#2022,#2023,#2024,#2025,#2026,#2027,#2028,
#2029,#2030,#2031,#2032,#2033,#2034,#2035,#2036,#2037,#2038,#2039,#2040,
#2041,#2042,#2043,#2044)) ;
#2261=AXIS2_PLACEMENT_3D('',#3218,#2617,#2618) ;
#2262=AXIS2_PLACEMENT_3D('',#3219,#2619,#2620) ;
#2263=AXIS2_PLACEMENT_3D('',#3221,#2621,#2622) ;
#2264=AXIS2_PLACEMENT_3D('',#3224,#2624,#2625) ;
#2265=AXIS2_PLACEMENT_3D('',#3225,#2626,#2627) ;
#2266=AXIS2_PLACEMENT_3D('',#3227,#2628,#2629) ;
#2267=AXIS2_PLACEMENT_3D('',#3230,#2631,#2632) ;
#2268=AXIS2_PLACEMENT_3D('',#3231,#2633,#2634) ;
#2269=AXIS2_PLACEMENT_3D('',#3233,#2635,#2636) ;
#2270=AXIS2_PLACEMENT_3D('',#3236,#2638,#2639) ;
#2271=AXIS2_PLACEMENT_3D('',#3237,#2640,#2641) ;
#2272=AXIS2_PLACEMENT_3D('',#3239,#2642,#2643) ;
#2273=AXIS2_PLACEMENT_3D('',#3242,#2645,#2646) ;
#2274=AXIS2_PLACEMENT_3D('',#3243,#2647,#2648) ;
#2275=AXIS2_PLACEMENT_3D('',#3245,#2649,#2650) ;
#2276=AXIS2_PLACEMENT_3D('',#3248,#2652,#2653) ;
#2277=AXIS2_PLACEMENT_3D('',#3249,#2654,#2655) ;
#2278=AXIS2_PLACEMENT_3D('',#3251,#2656,#2657) ;
#2279=AXIS2_PLACEMENT_3D('',#3254,#2659,#2660) ;
#2280=AXIS2_PLACEMENT_3D('',#3255,#2661,#2662) ;
#2281=AXIS2_PLACEMENT_3D('',#3257,#2663,#2664) ;
#2282=AXIS2_PLACEMENT_3D('',#3260,#2666,#2667) ;
#2283=AXIS2_PLACEMENT_3D('',#3261,#2668,#2669) ;
#2284=AXIS2_PLACEMENT_3D('',#3263,#2670,#2671) ;
#2285=AXIS2_PLACEMENT_3D('',#3266,#2673,#2674) ;
#2286=AXIS2_PLACEMENT_3D('',#3267,#2675,#2676) ;
#2287=AXIS2_PLACEMENT_3D('',#3269,#2677,#2678) ;
#2288=AXIS2_PLACEMENT_3D('',#3272,#2680,#2681) ;
#2289=AXIS2_PLACEMENT_3D('',#3273,#2682,#2683) ;
#2290=AXIS2_PLACEMENT_3D('',#3275,#2684,#2685) ;
#2291=AXIS2_PLACEMENT_3D('',#3278,#2687,#2688) ;
#2292=AXIS2_PLACEMENT_3D('',#3279,#2689,#2690) ;
#2293=AXIS2_PLACEMENT_3D('',#3281,#2691,#2692) ;
#2294=AXIS2_PLACEMENT_3D('',#3284,#2694,#2695) ;
#2295=AXIS2_PLACEMENT_3D('',#3285,#2696,#2697) ;
#2296=AXIS2_PLACEMENT_3D('',#3287,#2698,#2699) ;
#2297=AXIS2_PLACEMENT_3D('',#3290,#2701,#2702) ;
#2298=AXIS2_PLACEMENT_3D('',#3291,#2703,#2704) ;
#2299=AXIS2_PLACEMENT_3D('',#3293,#2705,#2706) ;
#2300=AXIS2_PLACEMENT_3D('',#3296,#2708,#2709) ;
#2301=AXIS2_PLACEMENT_3D('',#3297,#2710,#2711) ;
#2302=AXIS2_PLACEMENT_3D('',#3299,#2712,#2713) ;
#2303=AXIS2_PLACEMENT_3D('',#3302,#2715,#2716) ;
#2304=AXIS2_PLACEMENT_3D('',#3303,#2717,#2718) ;
#2305=AXIS2_PLACEMENT_3D('',#3305,#2719,#2720) ;
#2306=AXIS2_PLACEMENT_3D('',#3308,#2722,#2723) ;
#2307=AXIS2_PLACEMENT_3D('',#3309,#2724,#2725) ;
#2308=AXIS2_PLACEMENT_3D('',#3311,#2726,#2727) ;
#2309=AXIS2_PLACEMENT_3D('',#3314,#2729,#2730) ;
#2310=AXIS2_PLACEMENT_3D('',#3315,#2731,#2732) ;
#2311=AXIS2_PLACEMENT_3D('',#3317,#2733,#2734) ;
#2312=AXIS2_PLACEMENT_3D('',#3320,#2736,#2737) ;
#2313=AXIS2_PLACEMENT_3D('',#3321,#2738,#2739) ;
#2314=AXIS2_PLACEMENT_3D('',#3323,#2740,#2741) ;
#2315=AXIS2_PLACEMENT_3D('',#3326,#2743,#2744) ;
#2316=AXIS2_PLACEMENT_3D('',#3327,#2745,#2746) ;
#2317=AXIS2_PLACEMENT_3D('',#3329,#2747,#2748) ;
#2318=AXIS2_PLACEMENT_3D('',#3332,#2750,#2751) ;
#2319=AXIS2_PLACEMENT_3D('',#3333,#2752,#2753) ;
#2320=AXIS2_PLACEMENT_3D('',#3335,#2754,#2755) ;
#2321=AXIS2_PLACEMENT_3D('',#3338,#2757,#2758) ;
#2322=AXIS2_PLACEMENT_3D('',#3339,#2759,#2760) ;
#2323=AXIS2_PLACEMENT_3D('',#3341,#2761,#2762) ;
#2324=AXIS2_PLACEMENT_3D('',#3344,#2764,#2765) ;
#2325=AXIS2_PLACEMENT_3D('',#3345,#2766,#2767) ;
#2326=AXIS2_PLACEMENT_3D('',#3347,#2768,#2769) ;
#2327=AXIS2_PLACEMENT_3D('',#3350,#2771,#2772) ;
#2328=AXIS2_PLACEMENT_3D('',#3351,#2773,#2774) ;
#2329=AXIS2_PLACEMENT_3D('',#3376,#2787,#2788) ;
#2330=AXIS2_PLACEMENT_3D('',#3401,#2801,#2802) ;
#2331=AXIS2_PLACEMENT_3D('',#3404,#2805,#2806) ;
#2332=AXIS2_PLACEMENT_3D('',#3406,#2808,#2809) ;
#2333=AXIS2_PLACEMENT_3D('',#3408,#2811,#2812) ;
#2334=AXIS2_PLACEMENT_3D('',#3410,#2814,#2815) ;
#2335=AXIS2_PLACEMENT_3D('',#3412,#2817,#2818) ;
#2336=AXIS2_PLACEMENT_3D('',#3414,#2820,#2821) ;
#2337=AXIS2_PLACEMENT_3D('',#3416,#2823,#2824) ;
#2338=AXIS2_PLACEMENT_3D('',#3417,#2825,#2826) ;
#2339=AXIS2_PLACEMENT_3D('',#3420,#2829,#2830) ;
#2340=AXIS2_PLACEMENT_3D('',#3422,#2832,#2833) ;
#2341=AXIS2_PLACEMENT_3D('',#3424,#2835,#2836) ;
#2617=DIRECTION('axis',(0.,0.,1.)) ;
#2618=DIRECTION('refdir',(1.,0.,0.)) ;
#2619=DIRECTION('center_axis',(0.,-1.,0.)) ;
#2620=DIRECTION('ref_axis',(0.,0.,-1.)) ;
#2621=DIRECTION('center_axis',(0.,1.,0.)) ;
#2622=DIRECTION('ref_axis',(0.,0.,-1.)) ;
#2623=DIRECTION('',(0.,-1.,0.)) ;
#2624=DIRECTION('center_axis',(0.,1.,0.)) ;
#2625=DIRECTION('ref_axis',(0.,0.,-1.)) ;
#2626=DIRECTION('center_axis',(0.,-1.,0.)) ;
#2627=DIRECTION('ref_axis',(0.,0.,-1.)) ;
#2628=DIRECTION('center_axis',(0.,1.,0.)) ;
#2629=DIRECTION('ref_axis',(0.,0.,-1.)) ;
#2630=DIRECTION('',(0.,-1.,0.)) ;
#2631=DIRECTION('center_axis',(0.,1.,0.)) ;
#2632=DIRECTION('ref_axis',(0.,0.,-1.)) ;
#2633=DIRECTION('center_axis',(0.,-1.,0.)) ;
#2634=DIRECTION('ref_axis',(0.,0.,-1.)) ;
#2635=DIRECTION('center_axis',(0.,1.,0.)) ;
#2636=DIRECTION('ref_axis',(0.,0.,-1.)) ;
#2637=DIRECTION('',(0.,-1.,0.)) ;
#2638=DIRECTION('center_axis',(0.,1.,0.)) ;
#2639=DIRECTION('ref_axis',(0.,0.,-1.)) ;
#2640=DIRECTION('center_axis',(0.,-1.,0.)) ;
#2641=DIRECTION('ref_axis',(0.,0.,-1.)) ;
#2642=DIRECTION('center_axis',(0.,1.,0.)) ;
#2643=DIRECTION('ref_axis',(0.,0.,-1.)) ;
#2644=DIRECTION('',(0.,-1.,0.)) ;
#2645=DIRECTION('center_axis',(0.,1.,0.)) ;
#2646=DIRECTION('ref_axis',(0.,0.,-1.)) ;
#2647=DIRECTION('center_axis',(0.,-1.,0.)) ;
#2648=DIRECTION('ref_axis',(0.,0.,-1.)) ;
#2649=DIRECTION('center_axis',(0.,1.,0.)) ;
#2650=DIRECTION('ref_axis',(0.,0.,-1.)) ;
#2651=DIRECTION('',(0.,-1.,0.)) ;
#2652=DIRECTION('center_axis',(0.,1.,0.)) ;
#2653=DIRECTION('ref_axis',(0.,0.,-1.)) ;
#2654=DIRECTION('center_axis',(0.,-1.,0.)) ;
#2655=DIRECTION('ref_axis',(0.,0.,-1.)) ;
#2656=DIRECTION('center_axis',(0.,1.,0.)) ;
#2657=DIRECTION('ref_axis',(0.,0.,1.)) ;
#2658=DIRECTION('',(0.,-1.,0.)) ;
#2659=DIRECTION('center_axis',(0.,1.,0.)) ;
#2660=DIRECTION('ref_axis',(0.,0.,1.)) ;
#2661=DIRECTION('center_axis',(0.,-1.,0.)) ;
#2662=DIRECTION('ref_axis',(0.,0.,-1.)) ;
#2663=DIRECTION('center_axis',(0.,1.,0.)) ;
#2664=DIRECTION('ref_axis',(0.,0.,1.)) ;
#2665=DIRECTION('',(0.,-1.,0.)) ;
#2666=DIRECTION('center_axis',(0.,1.,0.)) ;
#2667=DIRECTION('ref_axis',(0.,0.,1.)) ;
#2668=DIRECTION('center_axis',(0.,-1.,0.)) ;
#2669=DIRECTION('ref_axis',(0.,0.,-1.)) ;
#2670=DIRECTION('center_axis',(0.,1.,0.)) ;
#2671=DIRECTION('ref_axis',(0.,0.,1.)) ;
#2672=DIRECTION('',(0.,-1.,0.)) ;
#2673=DIRECTION('center_axis',(0.,1.,0.)) ;
#2674=DIRECTION('ref_axis',(0.,0.,1.)) ;
#2675=DIRECTION('center_axis',(0.,-1.,0.)) ;
#2676=DIRECTION('ref_axis',(0.,0.,-1.)) ;
#2677=DIRECTION('center_axis',(0.,1.,0.)) ;
#2678=DIRECTION('ref_axis',(0.,0.,1.)) ;
#2679=DIRECTION('',(0.,-1.,0.)) ;
#2680=DIRECTION('center_axis',(0.,1.,0.)) ;
#2681=DIRECTION('ref_axis',(0.,0.,1.)) ;
#2682=DIRECTION('center_axis',(0.,-1.,0.)) ;
#2683=DIRECTION('ref_axis',(0.,0.,-1.)) ;
#2684=DIRECTION('center_axis',(0.,1.,0.)) ;
#2685=DIRECTION('ref_axis',(0.,0.,1.)) ;
#2686=DIRECTION('',(0.,-1.,0.)) ;
#2687=DIRECTION('center_axis',(0.,1.,0.)) ;
#2688=DIRECTION('ref_axis',(0.,0.,1.)) ;
#2689=DIRECTION('center_axis',(0.,-1.,0.)) ;
#2690=DIRECTION('ref_axis',(0.,0.,-1.)) ;
#2691=DIRECTION('center_axis',(0.,1.,0.)) ;
#2692=DIRECTION('ref_axis',(0.,0.,-1.)) ;
#2693=DIRECTION('',(0.,-1.,0.)) ;
#2694=DIRECTION('center_axis',(0.,1.,0.)) ;
#2695=DIRECTION('ref_axis',(0.,0.,-1.)) ;
#2696=DIRECTION('center_axis',(0.,-1.,0.)) ;
#2697=DIRECTION('ref_axis',(0.,0.,-1.)) ;
#2698=DIRECTION('center_axis',(0.,1.,0.)) ;
#2699=DIRECTION('ref_axis',(0.,0.,-1.)) ;
#2700=DIRECTION('',(0.,-1.,0.)) ;
#2701=DIRECTION('center_axis',(0.,1.,0.)) ;
#2702=DIRECTION('ref_axis',(0.,0.,-1.)) ;
#2703=DIRECTION('center_axis',(0.,-1.,0.)) ;
#2704=DIRECTION('ref_axis',(0.,0.,-1.)) ;
#2705=DIRECTION('center_axis',(0.,1.,0.)) ;
#2706=DIRECTION('ref_axis',(0.,0.,-1.)) ;
#2707=DIRECTION('',(0.,-1.,0.)) ;
#2708=DIRECTION('center_axis',(0.,1.,0.)) ;
#2709=DIRECTION('ref_axis',(0.,0.,-1.)) ;
#2710=DIRECTION('center_axis',(0.,-1.,0.)) ;
#2711=DIRECTION('ref_axis',(0.,0.,-1.)) ;
#2712=DIRECTION('center_axis',(0.,1.,0.)) ;
#2713=DIRECTION('ref_axis',(0.,0.,-1.)) ;
#2714=DIRECTION('',(0.,-1.,0.)) ;
#2715=DIRECTION('center_axis',(0.,1.,0.)) ;
#2716=DIRECTION('ref_axis',(0.,0.,-1.)) ;
#2717=DIRECTION('center_axis',(0.,-1.,0.)) ;
#2718=DIRECTION('ref_axis',(0.,0.,-1.)) ;
#2719=DIRECTION('center_axis',(0.,1.,0.)) ;
#2720=DIRECTION('ref_axis',(0.,0.,-1.)) ;
#2721=DIRECTION('',(0.,-1.,0.)) ;
#2722=DIRECTION('center_axis',(0.,1.,0.)) ;
#2723=DIRECTION('ref_axis',(0.,0.,-1.)) ;
#2724=DIRECTION('center_axis',(0.,-1.,0.)) ;
#2725=DIRECTION('ref_axis',(0.,0.,-1.)) ;
#2726=DIRECTION('center_axis',(0.,1.,0.)) ;
#2727=DIRECTION('ref_axis',(0.,0.,-1.)) ;
#2728=DIRECTION('',(0.,-1.,0.)) ;
#2729=DIRECTION('center_axis',(0.,1.,0.)) ;
#2730=DIRECTION('ref_axis',(0.,0.,-1.)) ;
#2731=DIRECTION('center_axis',(0.,-1.,0.)) ;
#2732=DIRECTION('ref_axis',(0.,0.,-1.)) ;
#2733=DIRECTION('center_axis',(0.,1.,0.)) ;
#2734=DIRECTION('ref_axis',(0.,0.,1.)) ;
#2735=DIRECTION('',(0.,-1.,0.)) ;
#2736=DIRECTION('center_axis',(0.,1.,0.)) ;
#2737=DIRECTION('ref_axis',(0.,0.,1.)) ;
#2738=DIRECTION('center_axis',(0.,-1.,0.)) ;
#2739=DIRECTION('ref_axis',(0.,0.,-1.)) ;
#2740=DIRECTION('center_axis',(0.,1.,0.)) ;
#2741=DIRECTION('ref_axis',(0.,0.,1.)) ;
#2742=DIRECTION('',(0.,-1.,0.)) ;
#2743=DIRECTION('center_axis',(0.,1.,0.)) ;
#2744=DIRECTION('ref_axis',(0.,0.,1.)) ;
#2745=DIRECTION('center_axis',(0.,-1.,0.)) ;
#2746=DIRECTION('ref_axis',(0.,0.,-1.)) ;
#2747=DIRECTION('center_axis',(0.,1.,0.)) ;
#2748=DIRECTION('ref_axis',(0.,0.,1.)) ;
#2749=DIRECTION('',(0.,-1.,0.)) ;
#2750=DIRECTION('center_axis',(0.,1.,0.)) ;
#2751=DIRECTION('ref_axis',(0.,0.,1.)) ;
#2752=DIRECTION('center_axis',(0.,-1.,0.)) ;
#2753=DIRECTION('ref_axis',(0.,0.,-1.)) ;
#2754=DIRECTION('center_axis',(0.,1.,0.)) ;
#2755=DIRECTION('ref_axis',(0.,0.,1.)) ;
#2756=DIRECTION('',(0.,-1.,0.)) ;
#2757=DIRECTION('center_axis',(0.,1.,0.)) ;
#2758=DIRECTION('ref_axis',(0.,0.,1.)) ;
#2759=DIRECTION('center_axis',(0.,-1.,0.)) ;
#2760=DIRECTION('ref_axis',(0.,0.,-1.)) ;
#2761=DIRECTION('center_axis',(0.,1.,0.)) ;
#2762=DIRECTION('ref_axis',(0.,0.,1.)) ;
#2763=DIRECTION('',(0.,-1.,0.)) ;
#2764=DIRECTION('center_axis',(0.,1.,0.)) ;
#2765=DIRECTION('ref_axis',(0.,0.,1.)) ;
#2766=DIRECTION('center_axis',(0.,-1.,0.)) ;
#2767=DIRECTION('ref_axis',(0.,0.,-1.)) ;
#2768=DIRECTION('center_axis',(0.,1.,0.)) ;
#2769=DIRECTION('ref_axis',(0.,0.,1.)) ;
#2770=DIRECTION('',(0.,-1.,0.)) ;
#2771=DIRECTION('center_axis',(0.,1.,0.)) ;
#2772=DIRECTION('ref_axis',(0.,0.,1.)) ;
#2773=DIRECTION('center_axis',(0.,1.,0.)) ;
#2774=DIRECTION('ref_axis',(0.,0.,1.)) ;
#2775=DIRECTION('',(0.,0.,1.)) ;
#2776=DIRECTION('',(0.707106781186546,0.,0.707106781186549)) ;
#2777=DIRECTION('',(1.,0.,0.)) ;
#2778=DIRECTION('',(0.707106781186549,0.,-0.707106781186546)) ;
#2779=DIRECTION('',(0.,0.,-1.)) ;
#2780=DIRECTION('',(-0.707106781186549,0.,-0.707106781186546)) ;
#2781=DIRECTION('',(-1.,0.,0.)) ;
#2782=DIRECTION('',(-0.707106781186546,0.,0.707106781186549)) ;
#2783=DIRECTION('',(-1.,0.,0.)) ;
#2784=DIRECTION('',(-2.46716227694479E-16,0.,-1.)) ;
#2785=DIRECTION('',(1.,0.,0.)) ;
#2786=DIRECTION('',(1.2335811384724E-16,0.,1.)) ;
#2787=DIRECTION('center_axis',(0.,1.,0.)) ;
#2788=DIRECTION('ref_axis',(0.,0.,1.)) ;
#2789=DIRECTION('',(0.,0.,1.)) ;
#2790=DIRECTION('',(-0.707106781186546,0.,0.707106781186549)) ;
#2791=DIRECTION('',(-1.,0.,0.)) ;
#2792=DIRECTION('',(-0.707106781186549,0.,-0.707106781186546)) ;
#2793=DIRECTION('',(0.,0.,-1.)) ;
#2794=DIRECTION('',(0.707106781186549,0.,-0.707106781186546)) ;
#2795=DIRECTION('',(1.,0.,0.)) ;
#2796=DIRECTION('',(0.707106781186546,0.,0.707106781186549)) ;
#2797=DIRECTION('',(-2.46716227694479E-16,0.,-1.)) ;
#2798=DIRECTION('',(-1.,0.,0.)) ;
#2799=DIRECTION('',(1.2335811384724E-16,0.,1.)) ;
#2800=DIRECTION('',(1.,0.,0.)) ;
#2801=DIRECTION('center_axis',(1.,0.,0.)) ;
#2802=DIRECTION('ref_axis',(0.,0.,-1.)) ;
#2803=DIRECTION('',(0.,-1.,0.)) ;
#2804=DIRECTION('',(0.,-1.,0.)) ;
#2805=DIRECTION('center_axis',(0.707106781186549,0.,-0.707106781186546)) ;
#2806=DIRECTION('ref_axis',(-0.707106781186546,0.,-0.707106781186549)) ;
#2807=DIRECTION('',(0.,-1.,0.)) ;
#2808=DIRECTION('center_axis',(0.,0.,-1.)) ;
#2809=DIRECTION('ref_axis',(-1.,0.,0.)) ;
#2810=DIRECTION('',(0.,-1.,0.)) ;
#2811=DIRECTION('center_axis',(-0.707106781186546,0.,-0.707106781186549)) ;
#2812=DIRECTION('ref_axis',(-0.707106781186549,0.,0.707106781186546)) ;
#2813=DIRECTION('',(0.,-1.,0.)) ;
#2814=DIRECTION('center_axis',(-1.,0.,0.)) ;
#2815=DIRECTION('ref_axis',(0.,0.,1.)) ;
#2816=DIRECTION('',(0.,-1.,0.)) ;
#2817=DIRECTION('center_axis',(-0.707106781186546,0.,0.707106781186549)) ;
#2818=DIRECTION('ref_axis',(0.707106781186549,0.,0.707106781186546)) ;
#2819=DIRECTION('',(0.,-1.,0.)) ;
#2820=DIRECTION('center_axis',(0.,0.,1.)) ;
#2821=DIRECTION('ref_axis',(1.,0.,0.)) ;
#2822=DIRECTION('',(0.,-1.,0.)) ;
#2823=DIRECTION('center_axis',(0.707106781186549,0.,0.707106781186546)) ;
#2824=DIRECTION('ref_axis',(0.707106781186546,0.,-0.707106781186549)) ;
#2825=DIRECTION('center_axis',(-1.,0.,2.46716227694479E-16)) ;
#2826=DIRECTION('ref_axis',(2.46716227694479E-16,0.,1.)) ;
#2827=DIRECTION('',(0.,-1.,0.)) ;
#2828=DIRECTION('',(0.,-1.,0.)) ;
#2829=DIRECTION('center_axis',(0.,0.,1.)) ;
#2830=DIRECTION('ref_axis',(1.,0.,0.)) ;
#2831=DIRECTION('',(0.,-1.,0.)) ;
#2832=DIRECTION('center_axis',(1.,0.,-1.2335811384724E-16)) ;
#2833=DIRECTION('ref_axis',(-1.2335811384724E-16,0.,-1.)) ;
#2834=DIRECTION('',(0.,-1.,0.)) ;
#2835=DIRECTION('center_axis',(0.,0.,-1.)) ;
#2836=DIRECTION('ref_axis',(-1.,0.,0.)) ;
#3218=CARTESIAN_POINT('',(0.,0.,0.)) ;
#3219=CARTESIAN_POINT('Origin',(300.2,560.,18.2500000000001)) ;
#3220=CARTESIAN_POINT('',(300.2,560.,23.7500000000001)) ;
#3221=CARTESIAN_POINT('Origin',(300.2,560.,18.2500000000001)) ;
#3222=CARTESIAN_POINT('',(300.2,550.,23.7500000000001)) ;
#3223=CARTESIAN_POINT('',(300.2,560.,23.7500000000001)) ;
#3224=CARTESIAN_POINT('Origin',(300.2,550.,18.2500000000001)) ;
#3225=CARTESIAN_POINT('Origin',(300.199999999999,560.,123.25)) ;
#3226=CARTESIAN_POINT('',(300.199999999999,560.,128.75)) ;
#3227=CARTESIAN_POINT('Origin',(300.199999999999,560.,123.25)) ;
#3228=CARTESIAN_POINT('',(300.199999999999,550.,128.75)) ;
#3229=CARTESIAN_POINT('',(300.199999999999,560.,128.75)) ;
#3230=CARTESIAN_POINT('Origin',(300.199999999999,550.,123.25)) ;
#3231=CARTESIAN_POINT('Origin',(300.199999999998,560.,228.25)) ;
#3232=CARTESIAN_POINT('',(300.199999999998,560.,233.75)) ;
#3233=CARTESIAN_POINT('Origin',(300.199999999998,560.,228.25)) ;
#3234=CARTESIAN_POINT('',(300.199999999998,550.,233.75)) ;
#3235=CARTESIAN_POINT('',(300.199999999998,560.,233.75)) ;
#3236=CARTESIAN_POINT('Origin',(300.199999999998,550.,228.25)) ;
#3237=CARTESIAN_POINT('Origin',(300.199999999997,560.,333.25)) ;
#3238=CARTESIAN_POINT('',(300.199999999997,560.,338.75)) ;
#3239=CARTESIAN_POINT('Origin',(300.199999999997,560.,333.25)) ;
#3240=CARTESIAN_POINT('',(300.199999999997,550.,338.75)) ;
#3241=CARTESIAN_POINT('',(300.199999999997,560.,338.75)) ;
#3242=CARTESIAN_POINT('Origin',(300.199999999997,550.,333.25)) ;
#3243=CARTESIAN_POINT('Origin',(300.199999999996,560.,438.25)) ;
#3244=CARTESIAN_POINT('',(300.199999999996,560.,443.75)) ;
#3245=CARTESIAN_POINT('Origin',(300.199999999996,560.,438.25)) ;
#3246=CARTESIAN_POINT('',(300.199999999996,550.,443.75)) ;
#3247=CARTESIAN_POINT('',(300.199999999996,560.,443.75)) ;
#3248=CARTESIAN_POINT('Origin',(300.199999999996,550.,438.25)) ;
#3249=CARTESIAN_POINT('Origin',(900.200000000004,560.,438.25)) ;
#3250=CARTESIAN_POINT('',(900.200000000004,560.,443.75)) ;
#3251=CARTESIAN_POINT('Origin',(900.200000000004,560.,438.25)) ;
#3252=CARTESIAN_POINT('',(900.200000000004,550.,443.75)) ;
#3253=CARTESIAN_POINT('',(900.200000000004,560.,443.75)) ;
#3254=CARTESIAN_POINT('Origin',(900.200000000004,550.,438.25)) ;
#3255=CARTESIAN_POINT('Origin',(900.200000000003,560.,333.25)) ;
#3256=CARTESIAN_POINT('',(900.200000000003,560.,338.75)) ;
#3257=CARTESIAN_POINT('Origin',(900.200000000003,560.,333.25)) ;
#3258=CARTESIAN_POINT('',(900.200000000003,550.,338.75)) ;
#3259=CARTESIAN_POINT('',(900.200000000003,560.,338.75)) ;
#3260=CARTESIAN_POINT('Origin',(900.200000000003,550.,333.25)) ;
#3261=CARTESIAN_POINT('Origin',(900.200000000002,560.,228.25)) ;
#3262=CARTESIAN_POINT('',(900.200000000002,560.,233.75)) ;
#3263=CARTESIAN_POINT('Origin',(900.200000000002,560.,228.25)) ;
#3264=CARTESIAN_POINT('',(900.200000000002,550.,233.75)) ;
#3265=CARTESIAN_POINT('',(900.200000000002,560.,233.75)) ;
#3266=CARTESIAN_POINT('Origin',(900.200000000002,550.,228.25)) ;
#3267=CARTESIAN_POINT('Origin',(900.200000000001,560.,123.25)) ;
#3268=CARTESIAN_POINT('',(900.200000000001,560.,128.75)) ;
#3269=CARTESIAN_POINT('Origin',(900.200000000001,560.,123.25)) ;
#3270=CARTESIAN_POINT('',(900.200000000001,550.,128.75)) ;
#3271=CARTESIAN_POINT('',(900.200000000001,560.,128.75)) ;
#3272=CARTESIAN_POINT('Origin',(900.200000000001,550.,123.25)) ;
#3273=CARTESIAN_POINT('Origin',(900.2,560.,18.2499999999999)) ;
#3274=CARTESIAN_POINT('',(900.2,560.,23.75)) ;
#3275=CARTESIAN_POINT('Origin',(900.2,560.,18.2499999999999)) ;
#3276=CARTESIAN_POINT('',(900.2,550.,23.75)) ;
#3277=CARTESIAN_POINT('',(900.2,560.,23.7499999999999)) ;
#3278=CARTESIAN_POINT('Origin',(900.2,550.,18.2499999999999)) ;
#3279=CARTESIAN_POINT('Origin',(350.2,560.,-16.7500000000003)) ;
#3280=CARTESIAN_POINT('',(350.2,560.,-11.2500000000003)) ;
#3281=CARTESIAN_POINT('Origin',(350.2,560.,-16.7500000000003)) ;
#3282=CARTESIAN_POINT('',(350.2,550.,-11.2500000000003)) ;
#3283=CARTESIAN_POINT('',(350.2,560.,-11.2500000000003)) ;
#3284=CARTESIAN_POINT('Origin',(350.2,550.,-16.7500000000003)) ;
#3285=CARTESIAN_POINT('Origin',(450.2,560.,-16.7500000000003)) ;
#3286=CARTESIAN_POINT('',(450.2,560.,-11.2500000000003)) ;
#3287=CARTESIAN_POINT('Origin',(450.2,560.,-16.7500000000003)) ;
#3288=CARTESIAN_POINT('',(450.2,550.,-11.2500000000003)) ;
#3289=CARTESIAN_POINT('',(450.2,560.,-11.2500000000003)) ;
#3290=CARTESIAN_POINT('Origin',(450.2,550.,-16.7500000000003)) ;
#3291=CARTESIAN_POINT('Origin',(550.2,560.,-16.7500000000003)) ;
#3292=CARTESIAN_POINT('',(550.2,560.,-11.2500000000003)) ;
#3293=CARTESIAN_POINT('Origin',(550.2,560.,-16.7500000000003)) ;
#3294=CARTESIAN_POINT('',(550.2,550.,-11.2500000000003)) ;
#3295=CARTESIAN_POINT('',(550.2,560.,-11.2500000000003)) ;
#3296=CARTESIAN_POINT('Origin',(550.2,550.,-16.7500000000003)) ;
#3297=CARTESIAN_POINT('Origin',(650.2,560.,-16.7500000000003)) ;
#3298=CARTESIAN_POINT('',(650.2,560.,-11.2500000000003)) ;
#3299=CARTESIAN_POINT('Origin',(650.2,560.,-16.7500000000003)) ;
#3300=CARTESIAN_POINT('',(650.2,550.,-11.2500000000003)) ;
#3301=CARTESIAN_POINT('',(650.2,560.,-11.2500000000003)) ;
#3302=CARTESIAN_POINT('Origin',(650.2,550.,-16.7500000000003)) ;
#3303=CARTESIAN_POINT('Origin',(750.2,560.,-16.7500000000003)) ;
#3304=CARTESIAN_POINT('',(750.2,560.,-11.2500000000003)) ;
#3305=CARTESIAN_POINT('Origin',(750.2,560.,-16.7500000000003)) ;
#3306=CARTESIAN_POINT('',(750.2,550.,-11.2500000000003)) ;
#3307=CARTESIAN_POINT('',(750.2,560.,-11.2500000000003)) ;
#3308=CARTESIAN_POINT('Origin',(750.2,550.,-16.7500000000003)) ;
#3309=CARTESIAN_POINT('Origin',(850.2,560.,-16.7500000000003)) ;
#3310=CARTESIAN_POINT('',(850.2,560.,-11.2500000000003)) ;
#3311=CARTESIAN_POINT('Origin',(850.2,560.,-16.7500000000003)) ;
#3312=CARTESIAN_POINT('',(850.2,550.,-11.2500000000003)) ;
#3313=CARTESIAN_POINT('',(850.2,560.,-11.2500000000003)) ;
#3314=CARTESIAN_POINT('Origin',(850.2,550.,-16.7500000000003)) ;
#3315=CARTESIAN_POINT('Origin',(850.2,560.,473.25)) ;
#3316=CARTESIAN_POINT('',(850.2,560.,478.75)) ;
#3317=CARTESIAN_POINT('Origin',(850.2,560.,473.25)) ;
#3318=CARTESIAN_POINT('',(850.2,550.,478.75)) ;
#3319=CARTESIAN_POINT('',(850.2,560.,478.75)) ;
#3320=CARTESIAN_POINT('Origin',(850.2,550.,473.25)) ;
#3321=CARTESIAN_POINT('Origin',(750.2,560.,473.25)) ;
#3322=CARTESIAN_POINT('',(750.2,560.,478.75)) ;
#3323=CARTESIAN_POINT('Origin',(750.2,560.,473.25)) ;
#3324=CARTESIAN_POINT('',(750.2,550.,478.75)) ;
#3325=CARTESIAN_POINT('',(750.2,560.,478.75)) ;
#3326=CARTESIAN_POINT('Origin',(750.2,550.,473.25)) ;
#3327=CARTESIAN_POINT('Origin',(650.2,560.,473.25)) ;
#3328=CARTESIAN_POINT('',(650.2,560.,478.75)) ;
#3329=CARTESIAN_POINT('Origin',(650.2,560.,473.25)) ;
#3330=CARTESIAN_POINT('',(650.2,550.,478.75)) ;
#3331=CARTESIAN_POINT('',(650.2,560.,478.75)) ;
#3332=CARTESIAN_POINT('Origin',(650.2,550.,473.25)) ;
#3333=CARTESIAN_POINT('Origin',(550.2,560.,473.25)) ;
#3334=CARTESIAN_POINT('',(550.2,560.,478.75)) ;
#3335=CARTESIAN_POINT('Origin',(550.2,560.,473.25)) ;
#3336=CARTESIAN_POINT('',(550.2,550.,478.75)) ;
#3337=CARTESIAN_POINT('',(550.2,560.,478.75)) ;
#3338=CARTESIAN_POINT('Origin',(550.2,550.,473.25)) ;
#3339=CARTESIAN_POINT('Origin',(450.2,560.,473.25)) ;
#3340=CARTESIAN_POINT('',(450.2,560.,478.75)) ;
#3341=CARTESIAN_POINT('Origin',(450.2,560.,473.25)) ;
#3342=CARTESIAN_POINT('',(450.2,550.,478.75)) ;
#3343=CARTESIAN_POINT('',(450.2,560.,478.75)) ;
#3344=CARTESIAN_POINT('Origin',(450.2,550.,473.25)) ;
#3345=CARTESIAN_POINT('Origin',(350.2,560.,473.25)) ;
#3346=CARTESIAN_POINT('',(350.2,560.,478.75)) ;
#3347=CARTESIAN_POINT('Origin',(350.2,560.,473.25)) ;
#3348=CARTESIAN_POINT('',(350.2,550.,478.75)) ;
#3349=CARTESIAN_POINT('',(350.2,560.,478.75)) ;
#3350=CARTESIAN_POINT('Origin',(350.2,550.,473.25)) ;
#3351=CARTESIAN_POINT('Origin',(600.2,560.,228.25)) ;
#3352=CARTESIAN_POINT('',(280.2,560.,-26.75)) ;
#3353=CARTESIAN_POINT('',(280.2,560.,483.25)) ;
#3354=CARTESIAN_POINT('',(280.2,560.,-26.75)) ;
#3355=CARTESIAN_POINT('',(290.2,560.,493.25)) ;
#3356=CARTESIAN_POINT('',(280.2,560.,483.25)) ;
#3357=CARTESIAN_POINT('',(910.2,560.,493.25)) ;
#3358=CARTESIAN_POINT('',(290.2,560.,493.25)) ;
#3359=CARTESIAN_POINT('',(920.2,560.,483.25)) ;
#3360=CARTESIAN_POINT('',(910.2,560.,493.25)) ;
#3361=CARTESIAN_POINT('',(920.2,560.,-26.7500000000001)) ;
#3362=CARTESIAN_POINT('',(920.2,560.,-26.7500000000001)) ;
#3363=CARTESIAN_POINT('',(910.2,560.,-36.7500000000001)) ;
#3364=CARTESIAN_POINT('',(910.2,560.,-36.7500000000001)) ;
#3365=CARTESIAN_POINT('',(290.2,560.,-36.7500000000001)) ;
#3366=CARTESIAN_POINT('',(290.2,560.,-36.7500000000001)) ;
#3367=CARTESIAN_POINT('',(290.2,560.,-36.7500000000001)) ;
#3368=CARTESIAN_POINT('',(880.2,560.,3.24999999999995)) ;
#3369=CARTESIAN_POINT('',(320.2,560.,3.24999999999995)) ;
#3370=CARTESIAN_POINT('',(320.2,560.,3.24999999999995)) ;
#3371=CARTESIAN_POINT('',(880.2,560.,453.25)) ;
#3372=CARTESIAN_POINT('',(880.2,560.,3.24999999999995)) ;
#3373=CARTESIAN_POINT('',(320.2,560.,453.25)) ;
#3374=CARTESIAN_POINT('',(320.2,560.,453.25)) ;
#3375=CARTESIAN_POINT('',(320.2,560.,3.24999999999995)) ;
#3376=CARTESIAN_POINT('Origin',(600.2,550.,228.25)) ;
#3377=CARTESIAN_POINT('',(280.2,550.,-26.75)) ;
#3378=CARTESIAN_POINT('',(280.2,550.,483.25)) ;
#3379=CARTESIAN_POINT('',(280.2,550.,-26.75)) ;
#3380=CARTESIAN_POINT('',(290.2,550.,-36.7500000000001)) ;
#3381=CARTESIAN_POINT('',(290.2,550.,-36.7500000000001)) ;
#3382=CARTESIAN_POINT('',(910.2,550.,-36.7500000000001)) ;
#3383=CARTESIAN_POINT('',(290.2,550.,-36.7500000000001)) ;
#3384=CARTESIAN_POINT('',(920.2,550.,-26.7500000000001)) ;
#3385=CARTESIAN_POINT('',(910.2,550.,-36.7500000000001)) ;
#3386=CARTESIAN_POINT('',(920.2,550.,483.25)) ;
#3387=CARTESIAN_POINT('',(920.2,550.,-26.7500000000001)) ;
#3388=CARTESIAN_POINT('',(910.2,550.,493.25)) ;
#3389=CARTESIAN_POINT('',(910.2,550.,493.25)) ;
#3390=CARTESIAN_POINT('',(290.2,550.,493.25)) ;
#3391=CARTESIAN_POINT('',(290.2,550.,493.25)) ;
#3392=CARTESIAN_POINT('',(280.2,550.,483.25)) ;
#3393=CARTESIAN_POINT('',(880.2,550.,453.25)) ;
#3394=CARTESIAN_POINT('',(880.2,550.,3.24999999999995)) ;
#3395=CARTESIAN_POINT('',(880.2,550.,3.24999999999995)) ;
#3396=CARTESIAN_POINT('',(320.2,550.,3.24999999999995)) ;
#3397=CARTESIAN_POINT('',(320.2,550.,3.24999999999995)) ;
#3398=CARTESIAN_POINT('',(320.2,550.,453.25)) ;
#3399=CARTESIAN_POINT('',(320.2,550.,3.24999999999995)) ;
#3400=CARTESIAN_POINT('',(320.2,550.,453.25)) ;
#3401=CARTESIAN_POINT('Origin',(280.2,560.,-26.75)) ;
#3402=CARTESIAN_POINT('',(280.2,560.,483.25)) ;
#3403=CARTESIAN_POINT('',(280.2,560.,-26.75)) ;
#3404=CARTESIAN_POINT('Origin',(280.2,560.,483.25)) ;
#3405=CARTESIAN_POINT('',(290.2,560.,493.25)) ;
#3406=CARTESIAN_POINT('Origin',(290.2,560.,493.25)) ;
#3407=CARTESIAN_POINT('',(910.2,560.,493.25)) ;
#3408=CARTESIAN_POINT('Origin',(910.2,560.,493.25)) ;
#3409=CARTESIAN_POINT('',(920.2,560.,483.25)) ;
#3410=CARTESIAN_POINT('Origin',(920.2,560.,-26.7500000000001)) ;
#3411=CARTESIAN_POINT('',(920.2,560.,-26.7500000000001)) ;
#3412=CARTESIAN_POINT('Origin',(910.2,560.,-36.7500000000001)) ;
#3413=CARTESIAN_POINT('',(910.2,560.,-36.7500000000001)) ;
#3414=CARTESIAN_POINT('Origin',(290.2,560.,-36.7500000000001)) ;
#3415=CARTESIAN_POINT('',(290.2,560.,-36.7500000000001)) ;
#3416=CARTESIAN_POINT('Origin',(290.2,560.,-36.7500000000001)) ;
#3417=CARTESIAN_POINT('Origin',(880.2,560.,3.24999999999995)) ;
#3418=CARTESIAN_POINT('',(880.2,560.,453.25)) ;
#3419=CARTESIAN_POINT('',(880.2,560.,3.24999999999995)) ;
#3420=CARTESIAN_POINT('Origin',(320.2,560.,3.24999999999995)) ;
#3421=CARTESIAN_POINT('',(320.2,560.,3.24999999999995)) ;
#3422=CARTESIAN_POINT('Origin',(320.2,560.,3.24999999999995)) ;
#3423=CARTESIAN_POINT('',(320.2,560.,453.25)) ;
#3424=CARTESIAN_POINT('Origin',(320.2,560.,453.25)) ;
#3603=UNCERTAINTY_MEASURE_WITH_UNIT(LENGTH_MEASURE(0.01),#3620,
'DISTANCE_ACCURACY_VALUE',
'Maximum model space distance between geometric entities at asserted c
onnectivities') ;
#3609=UNCERTAINTY_MEASURE_WITH_UNIT(LENGTH_MEASURE(0.01),#3620,
'DISTANCE_ACCURACY_VALUE',
'Maximum model space distance between geometric entities at asserted c
onnectivities') ;
#3613=(
GEOMETRIC_REPRESENTATION_CONTEXT(3)
GLOBAL_UNCERTAINTY_ASSIGNED_CONTEXT((#3603))
GLOBAL_UNIT_ASSIGNED_CONTEXT((#3620,#3622,#3623))
REPRESENTATION_CONTEXT('','3D')
) ;
#3619=(
GEOMETRIC_REPRESENTATION_CONTEXT(3)
GLOBAL_UNCERTAINTY_ASSIGNED_CONTEXT((#3609))
GLOBAL_UNIT_ASSIGNED_CONTEXT((#3620,#3622,#3623))
REPRESENTATION_CONTEXT('','3D')
) ;
#3620=(
LENGTH_UNIT()
NAMED_UNIT(*)
SI_UNIT(.MILLI.,.METRE.)
) ;
#3622=(
NAMED_UNIT(*)
PLANE_ANGLE_UNIT()
SI_UNIT($,.RADIAN.)
) ;
#3623=(
NAMED_UNIT(*)
SI_UNIT($,.STERADIAN.)
SOLID_ANGLE_UNIT()
) ;
#3627=SHAPE_DEFINITION_REPRESENTATION(#3636,#3653) ;
#3636=PRODUCT_DEFINITION_SHAPE('',$,#3663) ;
#3653=SHAPE_REPRESENTATION('',(#2261),#3613) ;
#3659=PRODUCT_DEFINITION_CONTEXT('part definition',#3688,'design') ;
#3663=PRODUCT_DEFINITION('Vent_Panel','Vent_Panel',#3672,#3659) ;
#3672=PRODUCT_DEFINITION_FORMATION('',$,#3693) ;
#3688=APPLICATION_CONTEXT(
'Core Data for Automotive Mechanical Design Process') ;
#3689=PRODUCT_CONTEXT('part definition',#3688,'mechanical') ;
#3693=PRODUCT('Vent_Panel','Vent_Panel',$,(#3689)) ;
#3700=PRESENTATION_STYLE_ASSIGNMENT((#3702)) ;
#3702=SURFACE_STYLE_USAGE(.BOTH.,#3704) ;
#3704=SURFACE_SIDE_STYLE('',(#3706)) ;
#3706=SURFACE_STYLE_FILL_AREA(#3708) ;
#3708=FILL_AREA_STYLE('Opaque(202,209,238)',(#3710)) ;
#3710=FILL_AREA_STYLE_COLOUR('Opaque(202,209,238)',#3712) ;
#3712=COLOUR_RGB('Opaque(202,209,238)', 0.09019608, 0.27058824, 0.51372549) ;
ENDSEC;
END-ISO-10303-21;
